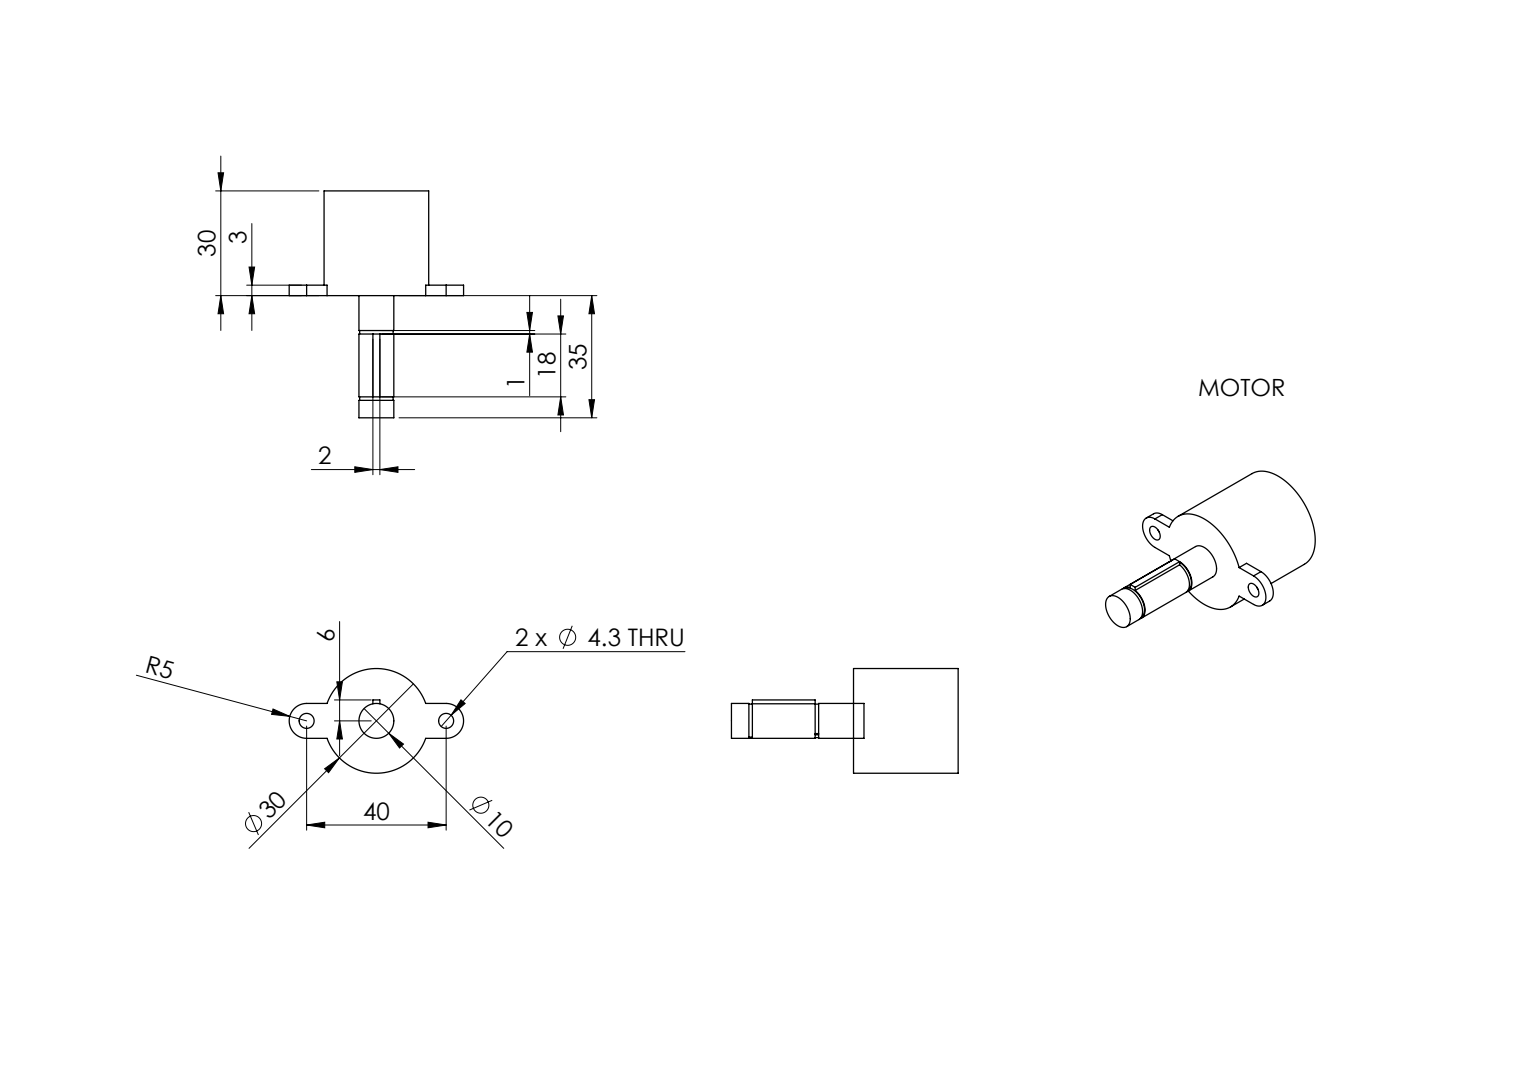
ISO-10303-21;
HEADER;
FILE_DESCRIPTION (('STEP AP214'),
    '1' );
FILE_NAME ('motor.step',
    '2026-10-31T03:44:21',
    ( '' ),
    ( '' ),
    'SwSTEP 2.0',
    'SolidWorks 2026',
    '' );
FILE_SCHEMA (( 'AUTOMOTIVE_DESIGN' ));
ENDSEC;

DATA;
#15=SURFACE_STYLE_USAGE ( .BOTH. , #11569 ) ;
#25=CARTESIAN_POINT ( 'NONE',  ( 5.000000000000003553, -20.00000000000000000, 9.999999999999998224 ) ) ;
#27=DIRECTION ( 'NONE',  ( -0.000000000000000000, -0.000000000000000000, -1.000000000000000000 ) ) ;
#44=CYLINDRICAL_SURFACE ( 'NONE', #13500, 4.799999999999999822 ) ;
#53=DIRECTION ( 'NONE',  ( -1.000000000000000000, 0.000000000000000000, 0.000000000000000000 ) ) ;
#55=CIRCLE ( 'NONE', #4760, 5.000000000000000888 ) ;
#73=CARTESIAN_POINT ( 'NONE',  ( 0.9183817310753816798, -24.91493387504114665, 15.00000000000000355 ) ) ;
#126=DIRECTION ( 'NONE',  ( -0.000000000000000000, -0.000000000000000000, -1.000000000000000000 ) ) ;
#134=ORIENTED_EDGE ( 'NONE', *, *, #5000, .T. ) ;
#135=DIRECTION ( 'NONE',  ( -9.710251638871371392E-17, -5.969973981896233748E-17, -1.000000000000000000 ) ) ;
#143=DIRECTION ( 'NONE',  ( -0.000000000000000000, -0.000000000000000000, -1.000000000000000000 ) ) ;
#149=DIRECTION ( 'NONE',  ( -0.6520673188974834833, 0.7581610723493047432, 1.805535875966851803E-17 ) ) ;
#153=VERTEX_POINT ( 'NONE', #25 ) ;
#166=CARTESIAN_POINT ( 'NONE',  ( 2.899426713160750069, -23.82535289025860337, -8.999999999999996447 ) ) ;
#171=DIRECTION ( 'NONE',  ( -0.000000000000000000, -0.000000000000000000, -1.000000000000000000 ) ) ;
#189=VERTEX_POINT ( 'NONE', #16887 ) ;
#191=ORIENTED_EDGE ( 'NONE', *, *, #16975, .F. ) ;
#195=EDGE_CURVE ( 'NONE', #14529, #9351, #3542, .T. ) ;
#218=CIRCLE ( 'NONE', #11155, 4.799999999999999822 ) ;
#226=VECTOR ( 'NONE', #4356, 1000.000000000000000 ) ;
#244=CARTESIAN_POINT ( 'NONE',  ( 22.14999999999999858, -20.00000000000000000, -20.00000000000000000 ) ) ;
#249=DIRECTION ( 'NONE',  ( -9.710251638871371392E-17, -5.969973981896233748E-17, -1.000000000000000000 ) ) ;
#257=DIRECTION ( 'NONE',  ( 0.1836763462126260738, -0.9829867750086873635, -1.521953536530129477E-22 ) ) ;
#284=ORIENTED_EDGE ( 'NONE', *, *, #7843, .F. ) ;
#301=EDGE_CURVE ( 'NONE', #4092, #18359, #6415, .T. ) ;
#302=EDGE_LOOP ( 'NONE', ( #1176, #3986, #11938, #3229 ) ) ;
#332=AXIS2_PLACEMENT_3D ( 'NONE', #14150, #12396, #6331 ) ;
#421=ORIENTED_EDGE ( 'NONE', *, *, #11100, .F. ) ;
#427=DIRECTION ( 'NONE',  ( -9.710251638871371392E-17, -5.969973981896233748E-17, -1.000000000000000000 ) ) ;
#449=CARTESIAN_POINT ( 'NONE',  ( 1.171083334267915221, -24.65495046420793201, 9.999999999999998224 ) ) ;
#461=ORIENTED_EDGE ( 'NONE', *, *, #12754, .F. ) ;
#464=VECTOR ( 'NONE', #12532, 1000.000000000000000 ) ;
#476=CARTESIAN_POINT ( 'NONE',  ( 2.449293598294706513E-15, -20.00000000000000000, -50.00000000000000000 ) ) ;
#480=CARTESIAN_POINT ( 'NONE',  ( 15.00000000000000178, -20.00000000000000000, -50.00000000000000000 ) ) ;
#484=ORIENTED_EDGE ( 'NONE', *, *, #4734, .T. ) ;
#531=CARTESIAN_POINT ( 'NONE',  ( 20.00000000000000000, -14.99999999999999289, -20.00000000000000000 ) ) ;
#541=ORIENTED_EDGE ( 'NONE', *, *, #9614, .T. ) ;
#547=AXIS2_PLACEMENT_3D ( 'NONE', #18765, #4147, #14614 ) ;
#556=ORIENTED_EDGE ( 'NONE', *, *, #7640, .F. ) ;
#557=VECTOR ( 'NONE', #8744, 1000.000000000000000 ) ;
#589=CYLINDRICAL_SURFACE ( 'NONE', #2546, 5.000000000000000888 ) ;
#603=LINE ( 'NONE', #2181, #4937 ) ;
#607=CYLINDRICAL_SURFACE ( 'NONE', #15492, 15.00000000000000000 ) ;
#614=CARTESIAN_POINT ( 'NONE',  ( 2.449293598294706513E-15, -20.00000000000000000, 15.00000000000000355 ) ) ;
#644=EDGE_CURVE ( 'NONE', #9042, #12835, #16688, .T. ) ;
#649=CIRCLE ( 'NONE', #7227, 5.000000000000007994 ) ;
#658=ADVANCED_FACE ( 'NONE', ( #13962 ), #8085, .T. ) ;
#664=CARTESIAN_POINT ( 'NONE',  ( 1.267864665261691752E-11, -20.00000000000000000, 9.999999999999998224 ) ) ;
#704=CIRCLE ( 'NONE', #1338, 5.000000000000000888 ) ;
#726=ORIENTED_EDGE ( 'NONE', *, *, #14827, .T. ) ;
#733=CARTESIAN_POINT ( 'NONE',  ( 2.899426713160750069, -23.82535289025860337, -8.999999999999996447 ) ) ;
#741=DIRECTION ( 'NONE',  ( 0.000000000000000000, 1.000000000000000000, 0.000000000000000000 ) ) ;
#781=ORIENTED_EDGE ( 'NONE', *, *, #10591, .F. ) ;
#787=EDGE_CURVE ( 'NONE', #6069, #5525, #6343, .T. ) ;
#805=LINE ( 'NONE', #17384, #2831 ) ;
#809=DIRECTION ( 'NONE',  ( 0.000000000000000000, 0.000000000000000000, -1.000000000000000000 ) ) ;
#839=DIRECTION ( 'NONE',  ( 0.000000000000000000, -0.000000000000000000, 1.000000000000000000 ) ) ;
#879=EDGE_LOOP ( 'NONE', ( #461, #556, #5752, #5214, #13460, #2512, #1411, #3266, #13006, #1930, #16328, #7538, #4298, #13725, #7198, #16875, #3831, #8695, #14190, #13668 ) ) ;
#883=EDGE_CURVE ( 'NONE', #9304, #15612, #704, .T. ) ;
#905=ADVANCED_FACE ( 'NONE', ( #9056 ), #10327, .F. ) ;
#909=AXIS2_PLACEMENT_3D ( 'NONE', #9474, #8004, #12326 ) ;
#926=VECTOR ( 'NONE', #18447, 1000.000000000000000 ) ;
#932=ORIENTED_EDGE ( 'NONE', *, *, #15552, .T. ) ;
#948=EDGE_LOOP ( 'NONE', ( #5660, #14767, #16075, #4087 ) ) ;
#953=EDGE_CURVE ( 'NONE', #5878, #5734, #2284, .T. ) ;
#967=DIRECTION ( 'NONE',  ( 9.858538378746663627E-23, -5.031452844637890958E-23, 1.000000000000000000 ) ) ;
#999=CARTESIAN_POINT ( 'NONE',  ( -4.999999999999998224, -20.00000000000000000, 15.00000000000000355 ) ) ;
#1006=ADVANCED_FACE ( 'NONE', ( #11896, #16716 ), #7399, .T. ) ;
#1036=ORIENTED_EDGE ( 'NONE', *, *, #11412, .T. ) ;
#1043=DIRECTION ( 'NONE',  ( 0.000000000000000000, 0.000000000000000000, -1.000000000000000000 ) ) ;
#1044=DIRECTION ( 'NONE',  ( -0.9697813467099857254, -0.2439756946365076173, 1.379242460255691792E-22 ) ) ;
#1056=VERTEX_POINT ( 'NONE', #15617 ) ;
#1065=EDGE_CURVE ( 'NONE', #10087, #17459, #7878, .T. ) ;
#1073=DIRECTION ( 'NONE',  ( 9.858538378746663627E-23, -5.031452844637890958E-23, 1.000000000000000000 ) ) ;
#1080=VERTEX_POINT ( 'NONE', #8056 ) ;
#1094=CARTESIAN_POINT ( 'NONE',  ( 5.000000000000003553, -20.00000000000000000, 9.000000000000000000 ) ) ;
#1096=VERTEX_POINT ( 'NONE', #9722 ) ;
#1107=CARTESIAN_POINT ( 'NONE',  ( -3.734041964264191549, -23.01611183630746638, -8.999999999999996447 ) ) ;
#1109=DIRECTION ( 'NONE',  ( 1.000000000000000000, 0.000000000000000000, 0.000000000000000000 ) ) ;
#1111=LINE ( 'NONE', #17781, #4763 ) ;
#1120=CARTESIAN_POINT ( 'NONE',  ( 2.449293598294706513E-15, -20.00000000000000000, -20.00000000000000000 ) ) ;
#1130=EDGE_CURVE ( 'NONE', #18302, #12106, #15719, .T. ) ;
#1132=DIRECTION ( 'NONE',  ( 0.000000000000000000, 0.000000000000000000, 1.000000000000000000 ) ) ;
#1152=ORIENTED_EDGE ( 'NONE', *, *, #9150, .T. ) ;
#1155=DIRECTION ( 'NONE',  ( -9.858538378746663627E-23, 5.031452844637890958E-23, -1.000000000000000000 ) ) ;
#1168=CARTESIAN_POINT ( 'NONE',  ( 1.267864665261691752E-11, -20.00000000000000000, 9.999999999999998224 ) ) ;
#1176=ORIENTED_EDGE ( 'NONE', *, *, #18527, .T. ) ;
#1179=EDGE_CURVE ( 'NONE', #8779, #4092, #13851, .T. ) ;
#1194=VECTOR ( 'NONE', #12290, 1000.000000000000000 ) ;
#1238=CIRCLE ( 'NONE', #3129, 5.000000000000000888 ) ;
#1241=ORIENTED_EDGE ( 'NONE', *, *, #11894, .T. ) ;
#1262=EDGE_CURVE ( 'NONE', #6920, #5143, #18873, .T. ) ;
#1296=( NAMED_UNIT ( * ) SI_UNIT ( $, .STERADIAN. ) SOLID_ANGLE_UNIT ( ) );
#1299=CARTESIAN_POINT ( 'NONE',  ( -20.00000000000000000, -19.99999999999999289, -20.00000000000000000 ) ) ;
#1301=DIRECTION ( 'NONE',  ( -0.9768494444668812671, -0.2139279384389642935, 0.000000000000000000 ) ) ;
#1321=VERTEX_POINT ( 'NONE', #1107 ) ;
#1338=AXIS2_PLACEMENT_3D ( 'NONE', #16043, #1132, #2717 ) ;
#1340=CARTESIAN_POINT ( 'NONE',  ( 2.449293598294706513E-15, -20.00000000000000000, 9.000000000000000000 ) ) ;
#1346=ORIENTED_EDGE ( 'NONE', *, *, #10591, .T. ) ;
#1361=ORIENTED_EDGE ( 'NONE', *, *, #9544, .T. ) ;
#1376=AXIS2_PLACEMENT_3D ( 'NONE', #10644, #15161, #18227 ) ;
#1386=( NAMED_UNIT ( * ) PLANE_ANGLE_UNIT ( ) SI_UNIT ( $, .RADIAN. ) );
#1411=ORIENTED_EDGE ( 'NONE', *, *, #17612, .T. ) ;
#1431=CARTESIAN_POINT ( 'NONE',  ( 1.219878473194463187, -24.84890673354692936, 9.000000000000000000 ) ) ;
#1433=VERTEX_POINT ( 'NONE', #19268 ) ;
#1440=CARTESIAN_POINT ( 'NONE',  ( 3.734041964264196434, -16.98388816369253362, -8.999999999999996447 ) ) ;
#1449=VECTOR ( 'NONE', #9677, 1000.000000000000000 ) ;
#1464=VERTEX_POINT ( 'NONE', #4636 ) ;
#1465=CIRCLE ( 'NONE', #3966, 5.000000000000000888 ) ;
#1515=LINE ( 'NONE', #10515, #14294 ) ;
#1537=DIRECTION ( 'NONE',  ( -9.710251638871371392E-17, -5.969973981896233748E-17, -1.000000000000000000 ) ) ;
#1540=EDGE_LOOP ( 'NONE', ( #1152, #15028, #8656, #5746 ) ) ;
#1552=AXIS2_PLACEMENT_3D ( 'NONE', #12885, #14449, #2511 ) ;
#1564=DIRECTION ( 'NONE',  ( -1.000000000000000000, 0.000000000000000000, 0.000000000000000000 ) ) ;
#1583=CIRCLE ( 'NONE', #332, 2.149999999999999023 ) ;
#1589=ORIENTED_EDGE ( 'NONE', *, *, #12157, .F. ) ;
#1620=EDGE_CURVE ( 'NONE', #6069, #8597, #7945, .T. ) ;
#1639=ORIENTED_EDGE ( 'NONE', *, *, #8427, .F. ) ;
#1640=EDGE_CURVE ( 'NONE', #7188, #13385, #11165, .T. ) ;
#1649=VERTEX_POINT ( 'NONE', #1788 ) ;
#1658=AXIS2_PLACEMENT_3D ( 'NONE', #6218, #16429, #16626 ) ;
#1684=ORIENTED_EDGE ( 'NONE', *, *, #3634, .F. ) ;
#1726=DIRECTION ( 'NONE',  ( -0.000000000000000000, -0.000000000000000000, -1.000000000000000000 ) ) ;
#1729=AXIS2_PLACEMENT_3D ( 'NONE', #5086, #9578, #3243 ) ;
#1788=CARTESIAN_POINT ( 'NONE',  ( -4.999999999999998224, -20.00000000000000000, -8.999999999999998224 ) ) ;
#1801=CIRCLE ( 'NONE', #19045, 15.00000000000000000 ) ;
#1822=LINE ( 'NONE', #7693, #18162 ) ;
#1874=AXIS2_PLACEMENT_3D ( 'NONE', #13952, #15437, #13862 ) ;
#1885=AXIS2_PLACEMENT_3D ( 'NONE', #2595, #11864, #19063 ) ;
#1898=CARTESIAN_POINT ( 'NONE',  ( -4.999999999999998224, -20.00000000000000000, 9.000000000000000000 ) ) ;
#1908=EDGE_CURVE ( 'NONE', #2621, #7384, #4316, .T. ) ;
#1925=CARTESIAN_POINT ( 'NONE',  ( -4.999999999999998224, -20.00000000000000000, 15.00000000000000355 ) ) ;
#1930=ORIENTED_EDGE ( 'NONE', *, *, #7858, .T. ) ;
#1983=CYLINDRICAL_SURFACE ( 'NONE', #3497, 5.000000000000000888 ) ;
#1994=DIRECTION ( 'NONE',  ( -1.000000000000000000, 0.000000000000000000, 0.000000000000000000 ) ) ;
#2014=ORIENTED_EDGE ( 'NONE', *, *, #18527, .F. ) ;
#2023=LINE ( 'NONE', #449, #17601 ) ;
#2049=EDGE_LOOP ( 'NONE', ( #1684, #9569, #5626, #12124, #5368, #18796, #18625, #17262 ) ) ;
#2056=CIRCLE ( 'NONE', #18350, 4.799999999999999822 ) ;
#2059=ORIENTED_EDGE ( 'NONE', *, *, #953, .F. ) ;
#2075=CARTESIAN_POINT ( 'NONE',  ( 2.449293598294706513E-15, -20.00000000000000000, 15.00000000000000355 ) ) ;
#2095=EDGE_CURVE ( 'NONE', #2791, #16221, #9204, .T. ) ;
#2097=CARTESIAN_POINT ( 'NONE',  ( -0.9999999999999976685, -20.00000000000000000, 8.999999999999998224 ) ) ;
#2114=DIRECTION ( 'NONE',  ( -9.710251638871371392E-17, -5.969973981896233748E-17, -1.000000000000000000 ) ) ;
#2117=CYLINDRICAL_SURFACE ( 'NONE', #15082, 2.149999999999999023 ) ;
#2131=ADVANCED_FACE ( 'NONE', ( #3523 ), #16968, .F. ) ;
#2139=( NAMED_UNIT ( * ) PLANE_ANGLE_UNIT ( ) SI_UNIT ( $, .RADIAN. ) );
#2141=ORIENTED_EDGE ( 'NONE', *, *, #15552, .F. ) ;
#2167=ORIENTED_EDGE ( 'NONE', *, *, #12021, .F. ) ;
#2170=CARTESIAN_POINT ( 'NONE',  ( 15.00000000000000178, -20.00000000000000000, -50.00000000000000000 ) ) ;
#2172=DIRECTION ( 'NONE',  ( 1.000000000000000000, 0.000000000000000000, 0.000000000000000000 ) ) ;
#2178=CIRCLE ( 'NONE', #2497, 4.800000000000000711 ) ;
#2181=CARTESIAN_POINT ( 'NONE',  ( 5.000000000000003553, -20.00000000000000000, 15.00000000000000355 ) ) ;
#2189=AXIS2_PLACEMENT_3D ( 'NONE', #14814, #14713, #1301 ) ;
#2193=DIRECTION ( 'NONE',  ( 0.000000000000000000, 0.000000000000000000, 1.000000000000000000 ) ) ;
#2208=EDGE_CURVE ( 'NONE', #17459, #7605, #2451, .T. ) ;
#2209=ORIENTED_EDGE ( 'NONE', *, *, #1620, .F. ) ;
#2246=VECTOR ( 'NONE', #6356, 1000.000000000000000 ) ;
#2254=VERTEX_POINT ( 'NONE', #5566 ) ;
#2281=DIRECTION ( 'NONE',  ( 0.000000000000000000, 0.000000000000000000, 1.000000000000000000 ) ) ;
#2284=CIRCLE ( 'NONE', #8215, 2.149999999999999023 ) ;
#2297=FACE_OUTER_BOUND ( 'NONE', #18445, .T. ) ;
#2341=EDGE_CURVE ( 'NONE', #1056, #14529, #13510, .T. ) ;
#2342=DIRECTION ( 'NONE',  ( 0.000000000000000000, 0.000000000000000000, -1.000000000000000000 ) ) ;
#2348=ORIENTED_EDGE ( 'NONE', *, *, #18323, .F. ) ;
#2355=CARTESIAN_POINT ( 'NONE',  ( 2.385244779468109755E-15, -20.00000000000000000, -9.999999999999994671 ) ) ;
#2370=AXIS2_PLACEMENT_3D ( 'NONE', #8722, #12053, #16478 ) ;
#2401=LINE ( 'NONE', #5416, #10995 ) ;
#2418=ORIENTED_EDGE ( 'NONE', *, *, #18926, .T. ) ;
#2426=PLANE ( 'NONE',  #11494 ) ;
#2431=VECTOR ( 'NONE', #5881, 1000.000000000000000 ) ;
#2451=LINE ( 'NONE', #2653, #1449 ) ;
#2453=VECTOR ( 'NONE', #15403, 999.9999999999998863 ) ;
#2497=AXIS2_PLACEMENT_3D ( 'NONE', #18498, #18305, #16731 ) ;
#2511=DIRECTION ( 'NONE',  ( 1.000000000000000000, -1.734723475976807341E-16, 0.000000000000000000 ) ) ;
#2512=ORIENTED_EDGE ( 'NONE', *, *, #12998, .T. ) ;
#2526=EDGE_CURVE ( 'NONE', #5878, #8101, #2401, .T. ) ;
#2546=AXIS2_PLACEMENT_3D ( 'NONE', #3628, #18454, #14567 ) ;
#2550=AXIS2_PLACEMENT_3D ( 'NONE', #3299, #15637, #15439 ) ;
#2553=LINE ( 'NONE', #14672, #17765 ) ;
#2556=FACE_OUTER_BOUND ( 'NONE', #16354, .T. ) ;
#2569=LINE ( 'NONE', #14496, #4883 ) ;
#2586=EDGE_CURVE ( 'NONE', #189, #17705, #1111, .T. ) ;
#2595=CARTESIAN_POINT ( 'NONE',  ( 1.267864665261691752E-11, -20.00000000000000000, 9.999999999999998224 ) ) ;
#2621=VERTEX_POINT ( 'NONE', #6983 ) ;
#2627=CARTESIAN_POINT ( 'NONE',  ( 3.129923130707922496, -23.63917314727666152, -8.999999999999996447 ) ) ;
#2650=CARTESIAN_POINT ( 'NONE',  ( 20.00000000000000000, -20.00000000000000000, -20.00000000000000000 ) ) ;
#2652=DIRECTION ( 'NONE',  ( -0.7779254092217071648, -0.6283566325640553840, 0.000000000000000000 ) ) ;
#2653=CARTESIAN_POINT ( 'NONE',  ( -1.000000000000000000, -14.00000000000000000, 8.999999999999998224 ) ) ;
#2683=VECTOR ( 'NONE', #17447, 1000.000000000000000 ) ;
#2687=CARTESIAN_POINT ( 'NONE',  ( 20.00000000000000000, -20.00000000000000000, -23.00000000000000000 ) ) ;
#2696=EDGE_CURVE ( 'NONE', #7605, #9351, #4641, .T. ) ;
#2707=DIRECTION ( 'NONE',  ( 0.000000000000000000, 0.000000000000000000, -1.000000000000000000 ) ) ;
#2712=CARTESIAN_POINT ( 'NONE',  ( -4.688877333428353111, -21.02685410450703074, 9.999999999999998224 ) ) ;
#2717=DIRECTION ( 'NONE',  ( 1.000000000000000000, 0.000000000000000000, 0.000000000000000000 ) ) ;
#2745=DIRECTION ( 'NONE',  ( -4.082155997157844188E-16, 1.000000000000000000, 0.000000000000000000 ) ) ;
#2763=EDGE_CURVE ( 'NONE', #12835, #6920, #3511, .T. ) ;
#2764=AXIS2_PLACEMENT_3D ( 'NONE', #9423, #9512, #6382 ) ;
#2771=CARTESIAN_POINT ( 'NONE',  ( 2.449293598294706513E-15, -20.00000000000000000, -23.00000000000000000 ) ) ;
#2773=VECTOR ( 'NONE', #14133, 1000.000000000000000 ) ;
#2775=LINE ( 'NONE', #17768, #7973 ) ;
#2777=CYLINDRICAL_SURFACE ( 'NONE', #1885, 4.800000000000000711 ) ;
#2791=VERTEX_POINT ( 'NONE', #2170 ) ;
#2831=VECTOR ( 'NONE', #18960, 1000.000000000000000 ) ;
#2834=FACE_OUTER_BOUND ( 'NONE', #7295, .T. ) ;
#2841=EDGE_CURVE ( 'NONE', #7251, #10053, #7325, .T. ) ;
#2856=UNCERTAINTY_MEASURE_WITH_UNIT (LENGTH_MEASURE( 1.000000000000000082E-05 ), #11966, 'distance_accuracy_value', 'NONE');
#2857=CARTESIAN_POINT ( 'NONE',  ( 4.688877333453708829, -18.97314589549297281, 9.999999999999998224 ) ) ;
#2871=CARTESIAN_POINT ( 'NONE',  ( 0.000000000000000000, 0.000000000000000000, 0.000000000000000000 ) ) ;
#2893=EDGE_LOOP ( 'NONE', ( #14519, #1241, #8781, #541, #15083, #16639, #1361, #2418, #6160, #17930, #16178, #3967 ) ) ;
#2961=EDGE_CURVE ( 'NONE', #10552, #3811, #14966, .T. ) ;
#2963=FILL_AREA_STYLE ('',( #16396 ) ) ;
#2992=DIRECTION ( 'NONE',  ( -4.082155997157844188E-16, 1.000000000000000000, 0.000000000000000000 ) ) ;
#2996=EDGE_CURVE ( 'NONE', #8876, #2621, #15399, .T. ) ;
#3026=DIRECTION ( 'NONE',  ( -1.000000000000000000, 0.000000000000000000, 0.000000000000000000 ) ) ;
#3029=ORIENTED_EDGE ( 'NONE', *, *, #7729, .T. ) ;
#3050=CLOSED_SHELL ( 'NONE', ( #11551, #12818, #12677, #16496, #16720, #7692, #5212, #9043, #16819, #4658, #7547, #13586, #5565, #10107, #11468, #16105, #7593, #15278, #14470, #2131, #1006, #14914, #5238, #17940, #13003, #905, #6926, #658, #10337, #18770, #8668, #8209, #4637, #10878, #8572, #15621, #16901, #15242, #8795, #15598 ) ) ;
#3097=AXIS2_PLACEMENT_3D ( 'NONE', #13122, #9094, #19329 ) ;
#3107=ORIENTED_EDGE ( 'NONE', *, *, #2341, .F. ) ;
#3125=LINE ( 'NONE', #15355, #8048 ) ;
#3128=AXIS2_PLACEMENT_3D ( 'NONE', #1120, #2707, #13075 ) ;
#3129=AXIS2_PLACEMENT_3D ( 'NONE', #1340, #7313, #10147 ) ;
#3134=ORIENTED_EDGE ( 'NONE', *, *, #15693, .T. ) ;
#3145=DIRECTION ( 'NONE',  ( -0.7779254092217071648, -0.6283566325640553840, 0.000000000000000000 ) ) ;
#3196=AXIS2_PLACEMENT_3D ( 'NONE', #10224, #4259, #4072 ) ;
#3200=VECTOR ( 'NONE', #2745, 1000.000000000000000 ) ;
#3204=ORIENTED_EDGE ( 'NONE', *, *, #4625, .F. ) ;
#3208=EDGE_LOOP ( 'NONE', ( #4399, #3539, #9450, #15588 ) ) ;
#3212=PLANE ( 'NONE',  #13485 ) ;
#3229=ORIENTED_EDGE ( 'NONE', *, *, #17743, .F. ) ;
#3240=LINE ( 'NONE', #12050, #13687 ) ;
#3243=DIRECTION ( 'NONE',  ( -0.7779254092217071648, -0.6283566325640553840, 1.130512422757410748E-16 ) ) ;
#3266=ORIENTED_EDGE ( 'NONE', *, *, #10585, .F. ) ;
#3278=CARTESIAN_POINT ( 'NONE',  ( 17.85000000000000142, -20.00000000000000000, -20.00000000000000000 ) ) ;
#3285=DIRECTION ( 'NONE',  ( -1.000000000000000000, 0.000000000000000000, -0.000000000000000000 ) ) ;
#3299=CARTESIAN_POINT ( 'NONE',  ( 2.449293598294706513E-15, -20.00000000000000000, -23.00000000000000000 ) ) ;
#3302=PLANE ( 'NONE',  #15384 ) ;
#3326=VERTEX_POINT ( 'NONE', #11798 ) ;
#3346=AXIS2_PLACEMENT_3D ( 'NONE', #614, #7962, #15717 ) ;
#3360=FACE_OUTER_BOUND ( 'NONE', #8105, .T. ) ;
#3369=ORIENTED_EDGE ( 'NONE', *, *, #14240, .T. ) ;
#3417=ORIENTED_EDGE ( 'NONE', *, *, #11894, .F. ) ;
#3422=AXIS2_PLACEMENT_3D ( 'NONE', #664, #16952, #15176 ) ;
#3447=VECTOR ( 'NONE', #15223, 1000.000000000000000 ) ;
#3475=DIRECTION ( 'NONE',  ( -0.000000000000000000, -0.000000000000000000, 1.000000000000000000 ) ) ;
#3494=VECTOR ( 'NONE', #257, 999.9999999999998863 ) ;
#3497=AXIS2_PLACEMENT_3D ( 'NONE', #2075, #14115, #9598 ) ;
#3511=CIRCLE ( 'NONE', #13533, 5.000000000000000888 ) ;
#3515=ORIENTED_EDGE ( 'NONE', *, *, #14193, .F. ) ;
#3523=FACE_OUTER_BOUND ( 'NONE', #11989, .T. ) ;
#3528=ORIENTED_EDGE ( 'NONE', *, *, #7944, .F. ) ;
#3539=ORIENTED_EDGE ( 'NONE', *, *, #10524, .F. ) ;
#3542=LINE ( 'NONE', #9314, #9848 ) ;
#3579=ORIENTED_EDGE ( 'NONE', *, *, #883, .T. ) ;
#3607=ORIENTED_EDGE ( 'NONE', *, *, #10362, .F. ) ;
#3628=CARTESIAN_POINT ( 'NONE',  ( 2.449293598294706513E-15, -20.00000000000000000, 15.00000000000000355 ) ) ;
#3634=EDGE_CURVE ( 'NONE', #1433, #2791, #19259, .T. ) ;
#3645=CARTESIAN_POINT ( 'NONE',  ( 1.000000000000000000, -14.00000000000000000, 8.999999999999998224 ) ) ;
#3647=CARTESIAN_POINT ( 'NONE',  ( 2.449293598294706513E-15, -20.00000000000000000, -50.00000000000000000 ) ) ;
#3656=FACE_OUTER_BOUND ( 'NONE', #1540, .T. ) ;
#3712=CARTESIAN_POINT ( 'NONE',  ( 2.449293598294706513E-15, -20.00000000000000000, 15.00000000000000355 ) ) ;
#3737=VECTOR ( 'NONE', #14659, 1000.000000000000000 ) ;
#3797=CARTESIAN_POINT ( 'NONE',  ( 2.482347295856823136E-15, -20.00000000000000000, -8.999999999999996447 ) ) ;
#3811=VERTEX_POINT ( 'NONE', #11480 ) ;
#3820=EDGE_CURVE ( 'NONE', #1464, #8101, #12968, .T. ) ;
#3829=CARTESIAN_POINT ( 'NONE',  ( 2.482347295856823136E-15, -20.00000000000000000, -8.999999999999996447 ) ) ;
#3831=ORIENTED_EDGE ( 'NONE', *, *, #9143, .F. ) ;
#3864=EDGE_LOOP ( 'NONE', ( #6325, #14684, #12211, #4511 ) ) ;
#3870=ORIENTED_EDGE ( 'NONE', *, *, #1130, .T. ) ;
#3891=EDGE_LOOP ( 'NONE', ( #12395, #17263 ) ) ;
#3911=CARTESIAN_POINT ( 'NONE',  ( 3.020236159542450949, -23.98474259401938014, 15.00000000000000355 ) ) ;
#3943=DIRECTION ( 'NONE',  ( -1.000000000000000000, 0.000000000000000000, 0.000000000000000000 ) ) ;
#3963=CARTESIAN_POINT ( 'NONE',  ( -1.000000000000000000, -14.00000000000000000, -9.000000000000001776 ) ) ;
#3966=AXIS2_PLACEMENT_3D ( 'NONE', #14131, #2193, #6784 ) ;
#3967=ORIENTED_EDGE ( 'NONE', *, *, #195, .T. ) ;
#3986=ORIENTED_EDGE ( 'NONE', *, *, #14771, .F. ) ;
#3991=FACE_OUTER_BOUND ( 'NONE', #16059, .T. ) ;
#4040=ORIENTED_EDGE ( 'NONE', *, *, #15055, .F. ) ;
#4050=EDGE_CURVE ( 'NONE', #1649, #1056, #16119, .T. ) ;
#4063=EDGE_LOOP ( 'NONE', ( #8392, #17053 ) ) ;
#4072=DIRECTION ( 'NONE',  ( -1.000000000000000000, 0.000000000000000000, 0.000000000000000000 ) ) ;
#4087=ORIENTED_EDGE ( 'NONE', *, *, #4050, .F. ) ;
#4092=VERTEX_POINT ( 'NONE', #18267 ) ;
#4147=DIRECTION ( 'NONE',  ( 0.000000000000000000, 0.000000000000000000, -1.000000000000000000 ) ) ;
#4212=CARTESIAN_POINT ( 'NONE',  ( 4.688877333453707941, -18.97314589549297281, 9.999999999999998224 ) ) ;
#4215=CARTESIAN_POINT ( 'NONE',  ( 0.9183817310753817909, -24.91493387504115020, 9.000000000000000000 ) ) ;
#4259=DIRECTION ( 'NONE',  ( -9.710251638871371392E-17, -5.969973981896233748E-17, -1.000000000000000000 ) ) ;
#4298=ORIENTED_EDGE ( 'NONE', *, *, #1908, .F. ) ;
#4316=LINE ( 'NONE', #10285, #11766 ) ;
#4325=( LENGTH_UNIT ( ) NAMED_UNIT ( * ) SI_UNIT ( .MILLI., .METRE. ) );
#4331=DIRECTION ( 'NONE',  ( -0.000000000000000000, -0.000000000000000000, 1.000000000000000000 ) ) ;
#4356=DIRECTION ( 'NONE',  ( -0.000000000000000000, -0.000000000000000000, 1.000000000000000000 ) ) ;
#4360=EDGE_CURVE ( 'NONE', #1080, #13316, #7668, .T. ) ;
#4364=FACE_OUTER_BOUND ( 'NONE', #302, .T. ) ;
#4382=EDGE_LOOP ( 'NONE', ( #17344, #13774 ) ) ;
#4387=VERTEX_POINT ( 'NONE', #4215 ) ;
#4399=ORIENTED_EDGE ( 'NONE', *, *, #2526, .F. ) ;
#4455=ORIENTED_EDGE ( 'NONE', *, *, #14348, .F. ) ;
#4457=DIRECTION ( 'NONE',  ( 0.000000000000000000, 0.000000000000000000, -1.000000000000000000 ) ) ;
#4508=DIRECTION ( 'NONE',  ( -0.000000000000000000, -0.000000000000000000, 1.000000000000000000 ) ) ;
#4511=ORIENTED_EDGE ( 'NONE', *, *, #2696, .T. ) ;
#4550=AXIS2_PLACEMENT_3D ( 'NONE', #18472, #249, #12663 ) ;
#4559=CARTESIAN_POINT ( 'NONE',  ( 5.000000000000003553, -20.00000000000000000, -20.00000000000000000 ) ) ;
#4589=CARTESIAN_POINT ( 'NONE',  ( -20.00000000000000000, -25.00000000000000000, -20.00000000000000000 ) ) ;
#4625=EDGE_CURVE ( 'NONE', #15442, #4903, #13987, .T. ) ;
#4636=CARTESIAN_POINT ( 'NONE',  ( -22.14999999999999858, -19.99999999999999289, -23.00000000000000000 ) ) ;
#4637=ADVANCED_FACE ( 'NONE', ( #4711 ), #18543, .F. ) ;
#4641=LINE ( 'NONE', #11876, #15387 ) ;
#4656=VECTOR ( 'NONE', #4508, 1000.000000000000000 ) ;
#4658=ADVANCED_FACE ( 'NONE', ( #2556 ), #11537, .T. ) ;
#4672=MECHANICAL_DESIGN_GEOMETRIC_PRESENTATION_REPRESENTATION('',(#4964),#8404);
#4711=FACE_OUTER_BOUND ( 'NONE', #9286, .T. ) ;
#4717=VECTOR ( 'NONE', #1537, 1000.000000000000000 ) ;
#4734=EDGE_CURVE ( 'NONE', #6996, #18140, #12051, .T. ) ;
#4749=EDGE_CURVE ( 'NONE', #18696, #18359, #18831, .T. ) ;
#4760=AXIS2_PLACEMENT_3D ( 'NONE', #11167, #2281, #16993 ) ;
#4763=VECTOR ( 'NONE', #17399, 1000.000000000000000 ) ;
#4765=CARTESIAN_POINT ( 'NONE',  ( 0.000000000000000000, 0.000000000000000000, -9.000000000000001776 ) ) ;
#4775=CARTESIAN_POINT ( 'NONE',  ( 0.8816464618332836567, -24.71833652004169934, 9.000000000000000000 ) ) ;
#4787=EDGE_LOOP ( 'NONE', ( #8005, #10366, #16026, #5421 ) ) ;
#4834=CARTESIAN_POINT ( 'NONE',  ( 15.00000000000000178, -20.00000000000000000, -23.00000000000000000 ) ) ;
#4836=EDGE_CURVE ( 'NONE', #12060, #13420, #17254, .T. ) ;
#4841=FACE_OUTER_BOUND ( 'NONE', #11042, .T. ) ;
#4863=CARTESIAN_POINT ( 'NONE',  ( 2.449293598294706513E-15, -20.00000000000000000, -8.999999999999998224 ) ) ;
#4883=VECTOR ( 'NONE', #14788, 999.9999999999998863 ) ;
#4885=( NAMED_UNIT ( * ) SI_UNIT ( $, .STERADIAN. ) SOLID_ANGLE_UNIT ( ) );
#4903=VERTEX_POINT ( 'NONE', #4589 ) ;
#4904=LINE ( 'NONE', #10871, #13097 ) ;
#4928=VERTEX_POINT ( 'NONE', #11638 ) ;
#4933=CARTESIAN_POINT ( 'NONE',  ( -4.999999999999998224, -20.00000000000000000, -9.999999999999994671 ) ) ;
#4937=VECTOR ( 'NONE', #10888, 1000.000000000000000 ) ;
#4944=DIRECTION ( 'NONE',  ( -1.000000000000000000, 0.000000000000000000, 0.000000000000000000 ) ) ;
#4964=STYLED_ITEM('',(#19482),#15206);
#4986=DIRECTION ( 'NONE',  ( -1.000000000000000000, 1.734723475976806848E-16, 0.000000000000000000 ) ) ;
#4992=AXIS2_PLACEMENT_3D ( 'NONE', #12281, #18281, #1994 ) ;
#5000=EDGE_CURVE ( 'NONE', #15442, #189, #17049, .T. ) ;
#5029=CARTESIAN_POINT ( 'NONE',  ( 2.482347295856823136E-15, -20.00000000000000000, -8.999999999999996447 ) ) ;
#5050=ORIENTED_EDGE ( 'NONE', *, *, #11929, .F. ) ;
#5073=VERTEX_POINT ( 'NONE', #15721 ) ;
#5086=CARTESIAN_POINT ( 'NONE',  ( 2.385244779468109755E-15, -20.00000000000000000, -9.999999999999994671 ) ) ;
#5088=CARTESIAN_POINT ( 'NONE',  ( -14.14213562373094568, -14.99999999999998757, -20.00000000000000000 ) ) ;
#5094=DIRECTION ( 'NONE',  ( -1.000000000000000000, 0.000000000000000000, 0.000000000000000000 ) ) ;
#5118=LINE ( 'NONE', #17097, #17763 ) ;
#5120=LINE ( 'NONE', #9434, #10842 ) ;
#5143=VERTEX_POINT ( 'NONE', #5220 ) ;
#5145=AXIS2_PLACEMENT_3D ( 'NONE', #17979, #27, #8742 ) ;
#5156=AXIS2_PLACEMENT_3D ( 'NONE', #10694, #12353, #11071 ) ;
#5166=CARTESIAN_POINT ( 'NONE',  ( 20.00000000000000000, -25.00000000000000711, -23.00000000000000000 ) ) ;
#5170=LINE ( 'NONE', #11142, #10219 ) ;
#5212=ADVANCED_FACE ( 'NONE', ( #17396 ), #17598, .T. ) ;
#5214=ORIENTED_EDGE ( 'NONE', *, *, #13247, .F. ) ;
#5220=CARTESIAN_POINT ( 'NONE',  ( 1.171083334267915221, -24.65495046420793201, 9.000000000000000000 ) ) ;
#5226=CIRCLE ( 'NONE', #547, 2.149999999999999023 ) ;
#5238=ADVANCED_FACE ( 'NONE', ( #14523 ), #15915, .F. ) ;
#5240=ORIENTED_EDGE ( 'NONE', *, *, #15055, .T. ) ;
#5275=AXIS2_PLACEMENT_3D ( 'NONE', #1168, #1073, #7042 ) ;
#5299=LINE ( 'NONE', #999, #11197 ) ;
#5307=CARTESIAN_POINT ( 'NONE',  ( 2.449293598294706513E-15, -20.00000000000000000, -20.00000000000000000 ) ) ;
#5324=DIRECTION ( 'NONE',  ( 0.000000000000000000, 0.000000000000000000, 1.000000000000000000 ) ) ;
#5339=ORIENTED_EDGE ( 'NONE', *, *, #2841, .F. ) ;
#5349=DIRECTION ( 'NONE',  ( -1.000000000000000000, 0.000000000000000000, 0.000000000000000000 ) ) ;
#5368=ORIENTED_EDGE ( 'NONE', *, *, #16233, .T. ) ;
#5390=CARTESIAN_POINT ( 'NONE',  ( 14.14213562373095101, -25.00000000000000711, -20.00000000000000000 ) ) ;
#5404=CARTESIAN_POINT ( 'NONE',  ( 2.449293598294706513E-15, -20.00000000000000000, 9.999999999999998224 ) ) ;
#5407=CARTESIAN_POINT ( 'NONE',  ( 2.449293598294706513E-15, -20.00000000000000000, -20.00000000000000000 ) ) ;
#5408=ORIENTED_EDGE ( 'NONE', *, *, #15044, .T. ) ;
#5416=CARTESIAN_POINT ( 'NONE',  ( -17.85000000000000142, -19.99999999999999289, -23.00000000000000000 ) ) ;
#5421=ORIENTED_EDGE ( 'NONE', *, *, #8050, .T. ) ;
#5443=LINE ( 'NONE', #11421, #17890 ) ;
#5495=DIRECTION ( 'NONE',  ( -1.000000000000000000, 0.000000000000000000, 0.000000000000000000 ) ) ;
#5525=VERTEX_POINT ( 'NONE', #18179 ) ;
#5554=ORIENTED_EDGE ( 'NONE', *, *, #3634, .T. ) ;
#5565=ADVANCED_FACE ( 'NONE', ( #12453 ), #1983, .T. ) ;
#5566=CARTESIAN_POINT ( 'NONE',  ( 14.14213562373095101, -25.00000000000000711, -23.00000000000000000 ) ) ;
#5577=PLANE ( 'NONE',  #10588 ) ;
#5599=EDGE_CURVE ( 'NONE', #7384, #9761, #55, .T. ) ;
#5624=AXIS2_PLACEMENT_3D ( 'NONE', #5404, #15905, #10996 ) ;
#5626=ORIENTED_EDGE ( 'NONE', *, *, #4360, .T. ) ;
#5650=CARTESIAN_POINT ( 'NONE',  ( 0.8816464618332836567, -24.71833652004169934, 9.999999999999998224 ) ) ;
#5660=ORIENTED_EDGE ( 'NONE', *, *, #17612, .F. ) ;
#5724=ORIENTED_EDGE ( 'NONE', *, *, #644, .T. ) ;
#5734=VERTEX_POINT ( 'NONE', #16185 ) ;
#5746=ORIENTED_EDGE ( 'NONE', *, *, #4625, .T. ) ;
#5750=DIRECTION ( 'NONE',  ( -9.858538378746663627E-23, 5.031452844637890958E-23, -1.000000000000000000 ) ) ;
#5752=ORIENTED_EDGE ( 'NONE', *, *, #8061, .T. ) ;
#5759=AXIS2_PLACEMENT_3D ( 'NONE', #8457, #11684, #7279 ) ;
#5760=DIRECTION ( 'NONE',  ( -0.000000000000000000, -0.000000000000000000, 1.000000000000000000 ) ) ;
#5798=DIRECTION ( 'NONE',  ( -0.000000000000000000, -0.000000000000000000, -1.000000000000000000 ) ) ;
#5841=ORIENTED_EDGE ( 'NONE', *, *, #15145, .F. ) ;
#5850=LINE ( 'NONE', #1440, #4717 ) ;
#5854=CARTESIAN_POINT ( 'NONE',  ( 2.449293598294706513E-15, -20.00000000000000000, -50.00000000000000000 ) ) ;
#5878=VERTEX_POINT ( 'NONE', #6085 ) ;
#5881=DIRECTION ( 'NONE',  ( -9.858538378746663627E-23, 5.031452844637890958E-23, -1.000000000000000000 ) ) ;
#5921=FACE_OUTER_BOUND ( 'NONE', #11880, .T. ) ;
#5922=ADVANCED_BREP_SHAPE_REPRESENTATION ( '', ( #15206, #10359 ), #13801 ) ;
#5935=DIRECTION ( 'NONE',  ( 0.000000000000000000, 0.000000000000000000, -1.000000000000000000 ) ) ;
#5962=DIRECTION ( 'NONE',  ( 0.000000000000000000, 0.000000000000000000, 1.000000000000000000 ) ) ;
#5975=CARTESIAN_POINT ( 'NONE',  ( 14.14213562373094923, -14.99999999999999112, -50.00000000000000000 ) ) ;
#5981=ORIENTED_EDGE ( 'NONE', *, *, #1262, .F. ) ;
#5983=ORIENTED_EDGE ( 'NONE', *, *, #11667, .F. ) ;
#6004=PRESENTATION_STYLE_ASSIGNMENT (( #15 ) ) ;
#6069=VERTEX_POINT ( 'NONE', #12534 ) ;
#6085=CARTESIAN_POINT ( 'NONE',  ( -17.85000000000000142, -19.99999999999999289, -20.00000000000000000 ) ) ;
#6154=VERTEX_POINT ( 'NONE', #5088 ) ;
#6160=ORIENTED_EDGE ( 'NONE', *, *, #10585, .T. ) ;
#6186=DIRECTION ( 'NONE',  ( -1.000000000000000000, 0.000000000000000000, 0.000000000000000000 ) ) ;
#6194=CIRCLE ( 'NONE', #9303, 2.149999999999999023 ) ;
#6210=DIRECTION ( 'NONE',  ( -9.710251638871371392E-17, -5.969973981896233748E-17, -1.000000000000000000 ) ) ;
#6218=CARTESIAN_POINT ( 'NONE',  ( 1.000000000000002442, -20.00000000000000000, 8.999999999999998224 ) ) ;
#6231=FACE_OUTER_BOUND ( 'NONE', #2049, .T. ) ;
#6237=LINE ( 'NONE', #4775, #3494 ) ;
#6255=ORIENTED_EDGE ( 'NONE', *, *, #2996, .T. ) ;
#6312=CARTESIAN_POINT ( 'NONE',  ( 20.00000000000000000, -14.99999999999999289, -23.00000000000000000 ) ) ;
#6325=ORIENTED_EDGE ( 'NONE', *, *, #195, .F. ) ;
#6331=DIRECTION ( 'NONE',  ( -1.000000000000000000, 0.000000000000000000, 0.000000000000000000 ) ) ;
#6343=CIRCLE ( 'NONE', #12284, 5.000000000000007994 ) ;
#6356=DIRECTION ( 'NONE',  ( -0.000000000000000000, -0.000000000000000000, -1.000000000000000000 ) ) ;
#6365=ORIENTED_EDGE ( 'NONE', *, *, #1262, .T. ) ;
#6382=DIRECTION ( 'NONE',  ( -0.9768494444668812671, -0.2139279384389642935, 0.000000000000000000 ) ) ;
#6400=CARTESIAN_POINT ( 'NONE',  ( -14.14213562373094746, -25.00000000000000000, -50.00000000000000000 ) ) ;
#6409=EDGE_LOOP ( 'NONE', ( #7699, #3579 ) ) ;
#6411=VERTEX_POINT ( 'NONE', #17738 ) ;
#6415=CIRCLE ( 'NONE', #5156, 2.149999999999999023 ) ;
#6470=AXIS2_PLACEMENT_3D ( 'NONE', #10421, #6210, #8953 ) ;
#6474=CIRCLE ( 'NONE', #16202, 4.799999999999999822 ) ;
#6487=CYLINDRICAL_SURFACE ( 'NONE', #3346, 5.000000000000000888 ) ;
#6514=DIRECTION ( 'NONE',  ( -0.2439756946365075896, 0.9697813467099857254, 1.610118993450814692E-22 ) ) ;
#6529=ORIENTED_EDGE ( 'NONE', *, *, #2526, .T. ) ;
#6533=CYLINDRICAL_SURFACE ( 'NONE', #3422, 4.800000000000000711 ) ;
#6548=CARTESIAN_POINT ( 'NONE',  ( -20.00000000000000000, -25.00000000000000000, -23.00000000000000000 ) ) ;
#6552=ORIENTED_EDGE ( 'NONE', *, *, #8309, .F. ) ;
#6553=VERTEX_POINT ( 'NONE', #10652 ) ;
#6562=FACE_OUTER_BOUND ( 'NONE', #11946, .T. ) ;
#6605=ORIENTED_EDGE ( 'NONE', *, *, #2208, .F. ) ;
#6616=CIRCLE ( 'NONE', #3196, 5.000000000000000888 ) ;
#6631=ORIENTED_EDGE ( 'NONE', *, *, #12754, .T. ) ;
#6635=VECTOR ( 'NONE', #12020, 1000.000000000000000 ) ;
#6639=ORIENTED_EDGE ( 'NONE', *, *, #787, .F. ) ;
#6709=CARTESIAN_POINT ( 'NONE',  ( -20.00000000000000000, -19.99999999999999289, -23.00000000000000000 ) ) ;
#6721=DIRECTION ( 'NONE',  ( -0.7779254092217071648, -0.6283566325640553840, 0.000000000000000000 ) ) ;
#6726=AXIS2_PLACEMENT_3D ( 'NONE', #2355, #9872, #2652 ) ;
#6728=DIRECTION ( 'NONE',  ( -0.7779254092217071648, -0.6283566325640553840, 0.000000000000000000 ) ) ;
#6738=DIRECTION ( 'NONE',  ( -0.000000000000000000, -0.000000000000000000, -1.000000000000000000 ) ) ;
#6754=EDGE_CURVE ( 'NONE', #12106, #4903, #5443, .T. ) ;
#6775=ORIENTED_EDGE ( 'NONE', *, *, #2841, .T. ) ;
#6784=DIRECTION ( 'NONE',  ( 1.000000000000000000, 0.000000000000000000, 0.000000000000000000 ) ) ;
#6798=AXIS2_PLACEMENT_3D ( 'NONE', #2627, #7305, #14746 ) ;
#6812=AXIS2_PLACEMENT_3D ( 'NONE', #15705, #10101, #5495 ) ;
#6821=ORIENTED_EDGE ( 'NONE', *, *, #2586, .T. ) ;
#6838=DIRECTION ( 'NONE',  ( -1.000000000000000000, 0.000000000000000000, 0.000000000000000000 ) ) ;
#6860=AXIS2_PLACEMENT_3D ( 'NONE', #14836, #4457, #14735 ) ;
#6868=DIRECTION ( 'NONE',  ( 1.000000000000000000, 0.000000000000000000, 0.000000000000000000 ) ) ;
#6891=LINE ( 'NONE', #12879, #18829 ) ;
#6910=CARTESIAN_POINT ( 'NONE',  ( 20.00000000000000000, -20.00000000000000000, -23.00000000000000000 ) ) ;
#6920=VERTEX_POINT ( 'NONE', #1431 ) ;
#6926=ADVANCED_FACE ( 'NONE', ( #11902 ), #17912, .T. ) ;
#6951=FACE_OUTER_BOUND ( 'NONE', #14837, .T. ) ;
#6957=CARTESIAN_POINT ( 'NONE',  ( -1.000000000000000000, -14.00000000000000000, 8.999999999999998224 ) ) ;
#6983=CARTESIAN_POINT ( 'NONE',  ( 5.000000000000003553, -20.00000000000000000, -9.999999999999994671 ) ) ;
#6996=VERTEX_POINT ( 'NONE', #16631 ) ;
#7001=DIRECTION ( 'NONE',  ( -9.858538378746663627E-23, 5.031452844637890958E-23, -1.000000000000000000 ) ) ;
#7042=DIRECTION ( 'NONE',  ( -0.9768494444668812671, -0.2139279384389642935, 0.000000000000000000 ) ) ;
#7064=VECTOR ( 'NONE', #9390, 1000.000000000000000 ) ;
#7067=ORIENTED_EDGE ( 'NONE', *, *, #12208, .F. ) ;
#7135=DIRECTION ( 'NONE',  ( 0.7969485188038759604, 0.6040472319084893016, -1.134471691914156900E-16 ) ) ;
#7144=VERTEX_POINT ( 'NONE', #12966 ) ;
#7153=AXIS2_PLACEMENT_3D ( 'NONE', #14687, #7438, #1564 ) ;
#7176=AXIS2_PLACEMENT_3D ( 'NONE', #19212, #1726, #4944 ) ;
#7188=VERTEX_POINT ( 'NONE', #17305 ) ;
#7197=LINE ( 'NONE', #2712, #11787 ) ;
#7198=ORIENTED_EDGE ( 'NONE', *, *, #17743, .T. ) ;
#7211=EDGE_CURVE ( 'NONE', #9761, #7384, #9415, .T. ) ;
#7220=EDGE_LOOP ( 'NONE', ( #18713, #3528, #18449, #12607, #8310, #11150, #9153, #1346 ) ) ;
#7227=AXIS2_PLACEMENT_3D ( 'NONE', #8759, #16325, #16618 ) ;
#7248=ORIENTED_EDGE ( 'NONE', *, *, #2696, .F. ) ;
#7251=VERTEX_POINT ( 'NONE', #8065 ) ;
#7266=CARTESIAN_POINT ( 'NONE',  ( 3.734041964264196878, -16.98388816369253362, -9.999999999999994671 ) ) ;
#7279=DIRECTION ( 'NONE',  ( 1.000000000000000000, -1.734723475976807341E-16, 0.000000000000000000 ) ) ;
#7295=EDGE_LOOP ( 'NONE', ( #18594, #12238, #18039, #19184 ) ) ;
#7305=DIRECTION ( 'NONE',  ( -0.7581610723493046322, -0.6520673188974834833, 1.125475972357111981E-16 ) ) ;
#7313=DIRECTION ( 'NONE',  ( -9.858538378746663627E-23, 5.031452844637890958E-23, -1.000000000000000000 ) ) ;
#7316=LINE ( 'NONE', #5650, #14988 ) ;
#7325=LINE ( 'NONE', #19220, #16044 ) ;
#7346=DIRECTION ( 'NONE',  ( 9.710251638871371392E-17, 5.969973981896233748E-17, 1.000000000000000000 ) ) ;
#7384=VERTEX_POINT ( 'NONE', #4559 ) ;
#7394=EDGE_LOOP ( 'NONE', ( #6639, #7439, #19080, #2167 ) ) ;
#7399=PLANE ( 'NONE',  #10713 ) ;
#7427=AXIS2_PLACEMENT_3D ( 'NONE', #8302, #967, #9962 ) ;
#7429=CARTESIAN_POINT ( 'NONE',  ( -20.00000000000000000, -19.99999999999999289, -23.00000000000000000 ) ) ;
#7438=DIRECTION ( 'NONE',  ( -9.858538378746663627E-23, 5.031452844637890958E-23, -1.000000000000000000 ) ) ;
#7439=ORIENTED_EDGE ( 'NONE', *, *, #1620, .T. ) ;
#7457=CARTESIAN_POINT ( 'NONE',  ( 2.449293598294706513E-15, -20.00000000000000000, 9.000000000000000000 ) ) ;
#7488=ORIENTED_EDGE ( 'NONE', *, *, #18257, .T. ) ;
#7524=DIRECTION ( 'NONE',  ( 0.000000000000000000, 0.000000000000000000, -1.000000000000000000 ) ) ;
#7538=ORIENTED_EDGE ( 'NONE', *, *, #7211, .T. ) ;
#7547=ADVANCED_FACE ( 'NONE', ( #2297 ), #6487, .T. ) ;
#7558=DIRECTION ( 'NONE',  ( -9.858538378746663627E-23, 5.031452844637890958E-23, -1.000000000000000000 ) ) ;
#7560=EDGE_LOOP ( 'NONE', ( #2059, #6529, #11689, #4455 ) ) ;
#7561=CARTESIAN_POINT ( 'NONE',  ( 5.000000000000003553, -20.00000000000000000, 15.00000000000000355 ) ) ;
#7583=CARTESIAN_POINT ( 'NONE',  ( 3.734041964264196878, -16.98388816369253362, -8.999999999999996447 ) ) ;
#7589=CARTESIAN_POINT ( 'NONE',  ( -20.00000000000000000, -19.99999999999999289, -20.00000000000000000 ) ) ;
#7593=ADVANCED_FACE ( 'NONE', ( #3656 ), #12669, .T. ) ;
#7602=EDGE_CURVE ( 'NONE', #3326, #9351, #5120, .T. ) ;
#7605=VERTEX_POINT ( 'NONE', #3645 ) ;
#7623=ORIENTED_EDGE ( 'NONE', *, *, #11758, .T. ) ;
#7640=EDGE_CURVE ( 'NONE', #15612, #9304, #1465, .T. ) ;
#7641=DIRECTION ( 'NONE',  ( -0.000000000000000000, -0.000000000000000000, -1.000000000000000000 ) ) ;
#7649=PLANE ( 'NONE',  #19062 ) ;
#7668=CIRCLE ( 'NONE', #2370, 15.00000000000000000 ) ;
#7681=DIRECTION ( 'NONE',  ( -1.000000000000000000, 0.000000000000000000, 0.000000000000000000 ) ) ;
#7692=ADVANCED_FACE ( 'NONE', ( #4841 ), #10802, .T. ) ;
#7693=CARTESIAN_POINT ( 'NONE',  ( 14.14213562373095101, -25.00000000000000711, -50.00000000000000000 ) ) ;
#7699=ORIENTED_EDGE ( 'NONE', *, *, #7640, .T. ) ;
#7716=ORIENTED_EDGE ( 'NONE', *, *, #8061, .F. ) ;
#7729=EDGE_CURVE ( 'NONE', #16659, #3811, #218, .T. ) ;
#7758=CARTESIAN_POINT ( 'NONE',  ( 2.449293598294706513E-15, -20.00000000000000000, -8.999999999999998224 ) ) ;
#7767=EDGE_CURVE ( 'NONE', #17357, #15934, #17296, .T. ) ;
#7798=ORIENTED_EDGE ( 'NONE', *, *, #1065, .T. ) ;
#7807=VECTOR ( 'NONE', #18303, 1000.000000000000000 ) ;
#7825=DIRECTION ( 'NONE',  ( 1.000000000000000000, -1.734723475976807341E-16, -0.000000000000000000 ) ) ;
#7843=EDGE_CURVE ( 'NONE', #18140, #16659, #6474, .T. ) ;
#7858=EDGE_CURVE ( 'NONE', #13420, #8876, #12424, .T. ) ;
#7866=VECTOR ( 'NONE', #13397, 1000.000000000000000 ) ;
#7874=DIRECTION ( 'NONE',  ( -0.000000000000000000, -0.000000000000000000, 1.000000000000000000 ) ) ;
#7878=LINE ( 'NONE', #2097, #2773 ) ;
#7887=ORIENTED_EDGE ( 'NONE', *, *, #8658, .F. ) ;
#7890=PLANE ( 'NONE',  #1874 ) ;
#7941=AXIS2_PLACEMENT_3D ( 'NONE', #8746, #17301, #1109 ) ;
#7944=EDGE_CURVE ( 'NONE', #2791, #1433, #13059, .T. ) ;
#7945=LINE ( 'NONE', #14113, #17784 ) ;
#7951=CYLINDRICAL_SURFACE ( 'NONE', #2764, 4.800000000000000711 ) ;
#7955=EDGE_CURVE ( 'NONE', #8262, #7251, #3240, .T. ) ;
#7960=CARTESIAN_POINT ( 'NONE',  ( -14.14213562373094568, -25.00000000000000000, -20.00000000000000000 ) ) ;
#7962=DIRECTION ( 'NONE',  ( -0.000000000000000000, -0.000000000000000000, -1.000000000000000000 ) ) ;
#7963=DIRECTION ( 'NONE',  ( -1.000000000000000000, 0.000000000000000000, 0.000000000000000000 ) ) ;
#7973=VECTOR ( 'NONE', #5798, 1000.000000000000000 ) ;
#7977=ORIENTED_EDGE ( 'NONE', *, *, #7767, .T. ) ;
#7990=CARTESIAN_POINT ( 'NONE',  ( 2.449293598294706513E-15, -20.00000000000000000, 9.000000000000000000 ) ) ;
#8004=DIRECTION ( 'NONE',  ( 0.000000000000000000, 0.000000000000000000, -1.000000000000000000 ) ) ;
#8005=ORIENTED_EDGE ( 'NONE', *, *, #7767, .F. ) ;
#8045=CARTESIAN_POINT ( 'NONE',  ( 1.000000000000000444, -15.10102051443364246, 9.000000000000000000 ) ) ;
#8047=DIRECTION ( 'NONE',  ( -1.000000000000000000, 0.000000000000000000, 0.000000000000000000 ) ) ;
#8048=VECTOR ( 'NONE', #171, 1000.000000000000000 ) ;
#8050=EDGE_CURVE ( 'NONE', #5143, #15934, #17460, .T. ) ;
#8056=CARTESIAN_POINT ( 'NONE',  ( -14.99999999999999822, -19.99999999999999645, -23.00000000000000000 ) ) ;
#8061=EDGE_CURVE ( 'NONE', #15612, #19390, #5170, .T. ) ;
#8065=CARTESIAN_POINT ( 'NONE',  ( 20.00000000000000000, -14.99999999999999289, -23.00000000000000000 ) ) ;
#8078=AXIS2_PLACEMENT_3D ( 'NONE', #10969, #16978, #5094 ) ;
#8085=PLANE ( 'NONE',  #15416 ) ;
#8101=VERTEX_POINT ( 'NONE', #8110 ) ;
#8105=EDGE_LOOP ( 'NONE', ( #8653, #7977, #11759, #17968 ) ) ;
#8110=CARTESIAN_POINT ( 'NONE',  ( -17.85000000000000142, -19.99999999999999289, -23.00000000000000000 ) ) ;
#8169=ORIENTED_EDGE ( 'NONE', *, *, #6754, .T. ) ;
#8209=ADVANCED_FACE ( 'NONE', ( #2834 ), #19320, .F. ) ;
#8215=AXIS2_PLACEMENT_3D ( 'NONE', #7589, #12191, #7681 ) ;
#8227=ORIENTED_EDGE ( 'NONE', *, *, #11434, .T. ) ;
#8229=DIRECTION ( 'NONE',  ( -1.000000000000000000, 0.000000000000000000, 0.000000000000000000 ) ) ;
#8251=CARTESIAN_POINT ( 'NONE',  ( -20.00000000000000000, -19.99999999999999289, -23.00000000000000000 ) ) ;
#8260=AXIS2_PLACEMENT_3D ( 'NONE', #7758, #9416, #9316 ) ;
#8262=VERTEX_POINT ( 'NONE', #19120 ) ;
#8265=ORIENTED_EDGE ( 'NONE', *, *, #16517, .T. ) ;
#8280=AXIS2_PLACEMENT_3D ( 'NONE', #17907, #143, #53 ) ;
#8302=CARTESIAN_POINT ( 'NONE',  ( 1.267864665251833278E-11, -20.00000000000000000, 9.000000000000000000 ) ) ;
#8308=EDGE_CURVE ( 'NONE', #6920, #4928, #2553, .T. ) ;
#8309=EDGE_CURVE ( 'NONE', #18696, #8779, #6194, .T. ) ;
#8310=ORIENTED_EDGE ( 'NONE', *, *, #15693, .F. ) ;
#8316=DIRECTION ( 'NONE',  ( -1.000000000000000000, 1.734723475976806848E-16, 0.000000000000000000 ) ) ;
#8362=FACE_OUTER_BOUND ( 'NONE', #11445, .T. ) ;
#8392=ORIENTED_EDGE ( 'NONE', *, *, #3820, .F. ) ;
#8404=( GEOMETRIC_REPRESENTATION_CONTEXT ( 3 ) GLOBAL_UNCERTAINTY_ASSIGNED_CONTEXT ( ( #9109 ) ) GLOBAL_UNIT_ASSIGNED_CONTEXT ( ( #18621, #2139, #4885 ) ) REPRESENTATION_CONTEXT ( 'NONE', 'WORKASPACE' ) );
#8415=ORIENTED_EDGE ( 'NONE', *, *, #301, .F. ) ;
#8427=EDGE_CURVE ( 'NONE', #9042, #3326, #3125, .T. ) ;
#8441=AXIS2_PLACEMENT_3D ( 'NONE', #2687, #4331, #8639 ) ;
#8457=CARTESIAN_POINT ( 'NONE',  ( 20.00000000000000000, -14.99999999999999289, -23.00000000000000000 ) ) ;
#8495=ORIENTED_EDGE ( 'NONE', *, *, #4360, .F. ) ;
#8506=CYLINDRICAL_SURFACE ( 'NONE', #9887, 15.00000000000000000 ) ;
#8514=DIRECTION ( 'NONE',  ( 0.000000000000000000, 0.000000000000000000, -1.000000000000000000 ) ) ;
#8516=CARTESIAN_POINT ( 'NONE',  ( 22.14999999999999858, -20.00000000000000000, -23.00000000000000000 ) ) ;
#8539=DIRECTION ( 'NONE',  ( -0.000000000000000000, -0.000000000000000000, -1.000000000000000000 ) ) ;
#8572=ADVANCED_FACE ( 'NONE', ( #9841 ), #2426, .F. ) ;
#8573=EDGE_LOOP ( 'NONE', ( #8415, #13227 ) ) ;
#8582=AXIS2_PLACEMENT_3D ( 'NONE', #7429, #7524, #3026 ) ;
#8597=VERTEX_POINT ( 'NONE', #16045 ) ;
#8616=ORIENTED_EDGE ( 'NONE', *, *, #15670, .F. ) ;
#8635=ORIENTED_EDGE ( 'NONE', *, *, #4734, .F. ) ;
#8639=DIRECTION ( 'NONE',  ( 1.000000000000000000, 0.000000000000000000, 0.000000000000000000 ) ) ;
#8651=APPLICATION_CONTEXT ( 'automotive_design' ) ;
#8653=ORIENTED_EDGE ( 'NONE', *, *, #13461, .F. ) ;
#8656=ORIENTED_EDGE ( 'NONE', *, *, #5000, .F. ) ;
#8658=EDGE_CURVE ( 'NONE', #16221, #2254, #18106, .T. ) ;
#8668=ADVANCED_FACE ( 'NONE', ( #4364 ), #18995, .F. ) ;
#8679=AXIS2_PLACEMENT_3D ( 'NONE', #476, #10671, #18248 ) ;
#8687=LINE ( 'NONE', #12010, #3737 ) ;
#8692=LINE ( 'NONE', #73, #15975 ) ;
#8695=ORIENTED_EDGE ( 'NONE', *, *, #2763, .T. ) ;
#8700=CARTESIAN_POINT ( 'NONE',  ( 2.899426713160750069, -23.82535289025860337, -8.999999999999996447 ) ) ;
#8722=CARTESIAN_POINT ( 'NONE',  ( 2.449293598294706513E-15, -20.00000000000000000, -23.00000000000000000 ) ) ;
#8730=DIRECTION ( 'NONE',  ( 1.000000000000000000, 0.000000000000000000, -0.000000000000000000 ) ) ;
#8735=CARTESIAN_POINT ( 'NONE',  ( 1.267864665261691752E-11, -20.00000000000000000, 9.999999999999998224 ) ) ;
#8742=DIRECTION ( 'NONE',  ( -1.000000000000000000, 0.000000000000000000, 0.000000000000000000 ) ) ;
#8744=DIRECTION ( 'NONE',  ( -0.2439756946365075896, 0.9697813467099857254, 1.610118993450814692E-22 ) ) ;
#8746=CARTESIAN_POINT ( 'NONE',  ( 20.00000000000000000, -20.00000000000000000, -23.00000000000000000 ) ) ;
#8759=CARTESIAN_POINT ( 'NONE',  ( 20.00000000000000000, -20.00000000000000000, -20.00000000000000000 ) ) ;
#8779=VERTEX_POINT ( 'NONE', #3278 ) ;
#8781=ORIENTED_EDGE ( 'NONE', *, *, #9024, .T. ) ;
#8795=ADVANCED_FACE ( 'NONE', ( #9158 ), #12192, .F. ) ;
#8814=LINE ( 'NONE', #10374, #9657 ) ;
#8833=DIRECTION ( 'NONE',  ( 0.000000000000000000, 0.000000000000000000, 1.000000000000000000 ) ) ;
#8834=DIRECTION ( 'NONE',  ( 0.000000000000000000, 0.000000000000000000, 1.000000000000000000 ) ) ;
#8858=FACE_BOUND ( 'NONE', #15980, .T. ) ;
#8876=VERTEX_POINT ( 'NONE', #4933 ) ;
#8902=LINE ( 'NONE', #5975, #4656 ) ;
#8953=DIRECTION ( 'NONE',  ( -1.000000000000000000, 0.000000000000000000, 0.000000000000000000 ) ) ;
#8971=ORIENTED_EDGE ( 'NONE', *, *, #8308, .F. ) ;
#8975=FACE_OUTER_BOUND ( 'NONE', #14631, .T. ) ;
#8983=CIRCLE ( 'NONE', #13362, 2.149999999999999023 ) ;
#9016=CARTESIAN_POINT ( 'NONE',  ( -4.688877333428352223, -21.02685410450703074, 9.999999999999998224 ) ) ;
#9022=CIRCLE ( 'NONE', #5275, 4.800000000000000711 ) ;
#9023=CARTESIAN_POINT ( 'NONE',  ( 2.482347295856823136E-15, -20.00000000000000000, -8.999999999999996447 ) ) ;
#9024=EDGE_CURVE ( 'NONE', #7144, #10315, #9220, .T. ) ;
#9042=VERTEX_POINT ( 'NONE', #8045 ) ;
#9043=ADVANCED_FACE ( 'NONE', ( #6231 ), #607, .T. ) ;
#9056=FACE_OUTER_BOUND ( 'NONE', #13804, .T. ) ;
#9064=LINE ( 'NONE', #531, #7807 ) ;
#9067=CYLINDRICAL_SURFACE ( 'NONE', #7176, 2.149999999999999023 ) ;
#9094=DIRECTION ( 'NONE',  ( -0.000000000000000000, -0.000000000000000000, -1.000000000000000000 ) ) ;
#9109=UNCERTAINTY_MEASURE_WITH_UNIT (LENGTH_MEASURE( 1.000000000000000082E-05 ), #18621, 'distance_accuracy_value', 'NONE');
#9143=EDGE_CURVE ( 'NONE', #12835, #7144, #2775, .T. ) ;
#9150=EDGE_CURVE ( 'NONE', #4903, #17705, #10172, .T. ) ;
#9153=ORIENTED_EDGE ( 'NONE', *, *, #1130, .F. ) ;
#9158=FACE_OUTER_BOUND ( 'NONE', #12033, .T. ) ;
#9176=EDGE_CURVE ( 'NONE', #6411, #17357, #11749, .T. ) ;
#9204=LINE ( 'NONE', #480, #7064 ) ;
#9209=DIRECTION ( 'NONE',  ( 9.858538378746663627E-23, -5.031452844637890958E-23, 1.000000000000000000 ) ) ;
#9212=CARTESIAN_POINT ( 'NONE',  ( 2.899426713160750069, -23.82535289025860337, -9.999999999999994671 ) ) ;
#9220=CIRCLE ( 'NONE', #4550, 5.000000000000000888 ) ;
#9221=DIRECTION ( 'NONE',  ( -0.000000000000000000, -0.000000000000000000, 1.000000000000000000 ) ) ;
#9234=LINE ( 'NONE', #12283, #3447 ) ;
#9251=CARTESIAN_POINT ( 'NONE',  ( 20.00000000000000000, -14.99999999999999289, -20.00000000000000000 ) ) ;
#9280=FACE_BOUND ( 'NONE', #4063, .T. ) ;
#9286=EDGE_LOOP ( 'NONE', ( #15930, #9459, #284, #8635, #2014, #5983, #11401, #16225 ) ) ;
#9290=LINE ( 'NONE', #15279, #2246 ) ;
#9303=AXIS2_PLACEMENT_3D ( 'NONE', #2650, #8514, #14484 ) ;
#9304=VERTEX_POINT ( 'NONE', #7561 ) ;
#9314=CARTESIAN_POINT ( 'NONE',  ( -1.000000000000000000, -14.00000000000000000, -9.000000000000001776 ) ) ;
#9316=DIRECTION ( 'NONE',  ( -1.000000000000000000, 0.000000000000000000, 0.000000000000000000 ) ) ;
#9327=ORIENTED_EDGE ( 'NONE', *, *, #1065, .F. ) ;
#9346=LINE ( 'NONE', #9251, #9981 ) ;
#9351=VERTEX_POINT ( 'NONE', #16690 ) ;
#9376=EDGE_LOOP ( 'NONE', ( #16985, #11950, #9828, #7067 ) ) ;
#9390=DIRECTION ( 'NONE',  ( -0.000000000000000000, -0.000000000000000000, 1.000000000000000000 ) ) ;
#9415=CIRCLE ( 'NONE', #15071, 5.000000000000000888 ) ;
#9416=DIRECTION ( 'NONE',  ( -9.710251638871371392E-17, -5.969973981896233748E-17, -1.000000000000000000 ) ) ;
#9423=CARTESIAN_POINT ( 'NONE',  ( 1.267864665261691752E-11, -20.00000000000000000, 9.999999999999998224 ) ) ;
#9434=CARTESIAN_POINT ( 'NONE',  ( 1.000000000000002442, -20.00000000000000000, -9.000000000000001776 ) ) ;
#9435=CARTESIAN_POINT ( 'NONE',  ( 2.449293598294706513E-15, -20.00000000000000000, -50.00000000000000000 ) ) ;
#9449=DIRECTION ( 'NONE',  ( 1.000000000000000000, -1.734723475976807341E-16, -0.000000000000000000 ) ) ;
#9450=ORIENTED_EDGE ( 'NONE', *, *, #14348, .T. ) ;
#9459=ORIENTED_EDGE ( 'NONE', *, *, #7729, .F. ) ;
#9474=CARTESIAN_POINT ( 'NONE',  ( 20.00000000000000000, -20.00000000000000000, -20.00000000000000000 ) ) ;
#9478=LINE ( 'NONE', #5166, #10046 ) ;
#9492=DIRECTION ( 'NONE',  ( -0.000000000000000000, -0.000000000000000000, -1.000000000000000000 ) ) ;
#9512=DIRECTION ( 'NONE',  ( -9.858538378746663627E-23, 5.031452844637890958E-23, -1.000000000000000000 ) ) ;
#9526=DIRECTION ( 'NONE',  ( -0.7779254092217071648, -0.6283566325640553840, 0.000000000000000000 ) ) ;
#9544=EDGE_CURVE ( 'NONE', #1321, #10552, #2056, .T. ) ;
#9569=ORIENTED_EDGE ( 'NONE', *, *, #18283, .T. ) ;
#9572=ORIENTED_EDGE ( 'NONE', *, *, #883, .F. ) ;
#9578=DIRECTION ( 'NONE',  ( -9.710251638871371392E-17, -5.969973981896234981E-17, -1.000000000000000000 ) ) ;
#9589=PLANE ( 'NONE',  #13778 ) ;
#9598=DIRECTION ( 'NONE',  ( -1.000000000000000000, 0.000000000000000000, 0.000000000000000000 ) ) ;
#9612=AXIS2_PLACEMENT_3D ( 'NONE', #10328, #14548, #12988 ) ;
#9614=EDGE_CURVE ( 'NONE', #10315, #5073, #2569, .T. ) ;
#9634=EDGE_LOOP ( 'NONE', ( #6365, #12125, #14607, #8971 ) ) ;
#9657=VECTOR ( 'NONE', #14786, 1000.000000000000000 ) ;
#9663=DIRECTION ( 'NONE',  ( 9.710251638871371392E-17, 5.969973981896233748E-17, 1.000000000000000000 ) ) ;
#9673=DIRECTION ( 'NONE',  ( -0.000000000000000000, -0.000000000000000000, -1.000000000000000000 ) ) ;
#9677=DIRECTION ( 'NONE',  ( 1.000000000000000000, 0.000000000000000000, 0.000000000000000000 ) ) ;
#9678=AXIS2_PLACEMENT_3D ( 'NONE', #3797, #11514, #6721 ) ;
#9708=ORIENTED_EDGE ( 'NONE', *, *, #11929, .T. ) ;
#9716=COLOUR_RGB ( '',0.8941176470588234615, 0.8941176470588234615, 0.8941176470588234615 ) ;
#9722=CARTESIAN_POINT ( 'NONE',  ( 20.00000000000000000, -25.00000000000000711, -20.00000000000000000 ) ) ;
#9761=VERTEX_POINT ( 'NONE', #10562 ) ;
#9770=CARTESIAN_POINT ( 'NONE',  ( 2.482347295856823136E-15, -20.00000000000000000, -8.999999999999996447 ) ) ;
#9773=DIRECTION ( 'NONE',  ( 1.000000000000000000, 0.000000000000000000, 0.000000000000000000 ) ) ;
#9790=DIRECTION ( 'NONE',  ( -0.7779254092217071648, -0.6283566325640553840, 0.000000000000000000 ) ) ;
#9828=ORIENTED_EDGE ( 'NONE', *, *, #7843, .T. ) ;
#9841=FACE_OUTER_BOUND ( 'NONE', #9634, .T. ) ;
#9848=VECTOR ( 'NONE', #2172, 1000.000000000000000 ) ;
#9861=CARTESIAN_POINT ( 'NONE',  ( 2.449293598294706513E-15, -20.00000000000000000, -50.00000000000000000 ) ) ;
#9872=DIRECTION ( 'NONE',  ( 9.710251638871371392E-17, 5.969973981896233748E-17, 1.000000000000000000 ) ) ;
#9883=CARTESIAN_POINT ( 'NONE',  ( 20.00000000000000000, -25.00000000000000711, -23.00000000000000000 ) ) ;
#9887=AXIS2_PLACEMENT_3D ( 'NONE', #9861, #17638, #9773 ) ;
#9898=CARTESIAN_POINT ( 'NONE',  ( -4.999999999999998224, -20.00000000000000000, 9.999999999999998224 ) ) ;
#9912=AXIS2_PLACEMENT_3D ( 'NONE', #8700, #7135, #13113 ) ;
#9919=DIRECTION ( 'NONE',  ( -0.000000000000000000, -0.000000000000000000, -1.000000000000000000 ) ) ;
#9946=CARTESIAN_POINT ( 'NONE',  ( -14.14213562373094746, -25.00000000000000000, -23.00000000000000000 ) ) ;
#9962=DIRECTION ( 'NONE',  ( -0.9768494444668812671, -0.2139279384389642935, 0.000000000000000000 ) ) ;
#9981=VECTOR ( 'NONE', #9449, 1000.000000000000000 ) ;
#9996=CIRCLE ( 'NONE', #4992, 2.149999999999999023 ) ;
#10046=VECTOR ( 'NONE', #17146, 1000.000000000000000 ) ;
#10051=CARTESIAN_POINT ( 'NONE',  ( 22.14999999999999858, -20.00000000000000000, -23.00000000000000000 ) ) ;
#10053=VERTEX_POINT ( 'NONE', #15766 ) ;
#10063=DIRECTION ( 'NONE',  ( -1.545477659731174253E-22, 3.805888647522192075E-23, -1.000000000000000000 ) ) ;
#10087=VERTEX_POINT ( 'NONE', #11719 ) ;
#10089=PRODUCT_DEFINITION ( 'UNKNOWN', '', #16398, #11655 ) ;
#10101=DIRECTION ( 'NONE',  ( -0.000000000000000000, -0.000000000000000000, -1.000000000000000000 ) ) ;
#10102=SHAPE_REPRESENTATION_RELATIONSHIP ( 'NONE' , 'NONE' ,  #19357, #5922 ) ;
#10107=ADVANCED_FACE ( 'NONE', ( #19013 ), #8506, .T. ) ;
#10147=DIRECTION ( 'NONE',  ( -1.000000000000000000, 0.000000000000000000, 0.000000000000000000 ) ) ;
#10172=CIRCLE ( 'NONE', #16156, 5.000000000000007994 ) ;
#10219=VECTOR ( 'NONE', #9673, 1000.000000000000000 ) ;
#10224=CARTESIAN_POINT ( 'NONE',  ( 2.449293598294706513E-15, -20.00000000000000000, -9.999999999999994671 ) ) ;
#10285=CARTESIAN_POINT ( 'NONE',  ( 5.000000000000003553, -20.00000000000000000, 15.00000000000000355 ) ) ;
#10295=ORIENTED_EDGE ( 'NONE', *, *, #1179, .T. ) ;
#10315=VERTEX_POINT ( 'NONE', #11916 ) ;
#10318=DIRECTION ( 'NONE',  ( -0.7779254092217071648, -0.6283566325640553840, 0.000000000000000000 ) ) ;
#10327=PLANE ( 'NONE',  #1658 ) ;
#10328=CARTESIAN_POINT ( 'NONE',  ( 2.449293598294706513E-15, -20.00000000000000000, -23.00000000000000000 ) ) ;
#10337=ADVANCED_FACE ( 'NONE', ( #8975 ), #3212, .F. ) ;
#10356=CARTESIAN_POINT ( 'NONE',  ( 2.449293598294706513E-15, -20.00000000000000000, 9.000000000000000000 ) ) ;
#10359=AXIS2_PLACEMENT_3D ( 'NONE', #2871, #8834, #16191 ) ;
#10362=EDGE_CURVE ( 'NONE', #11836, #18140, #5850, .T. ) ;
#10366=ORIENTED_EDGE ( 'NONE', *, *, #9176, .F. ) ;
#10374=CARTESIAN_POINT ( 'NONE',  ( 20.00000000000000000, -25.00000000000000711, -23.00000000000000000 ) ) ;
#10421=CARTESIAN_POINT ( 'NONE',  ( 2.449293598294706513E-15, -20.00000000000000000, -8.999999999999998224 ) ) ;
#10487=FACE_OUTER_BOUND ( 'NONE', #6409, .T. ) ;
#10492=CYLINDRICAL_SURFACE ( 'NONE', #16302, 4.799999999999999822 ) ;
#10515=CARTESIAN_POINT ( 'NONE',  ( 1.000000000000002442, -20.00000000000000000, 8.999999999999998224 ) ) ;
#10524=EDGE_CURVE ( 'NONE', #5734, #5878, #1583, .T. ) ;
#10542=CIRCLE ( 'NONE', #6470, 5.000000000000000888 ) ;
#10552=VERTEX_POINT ( 'NONE', #733 ) ;
#10562=CARTESIAN_POINT ( 'NONE',  ( -4.999999999999998224, -20.00000000000000000, -20.00000000000000000 ) ) ;
#10585=EDGE_CURVE ( 'NONE', #12060, #1649, #11904, .T. ) ;
#10588=AXIS2_PLACEMENT_3D ( 'NONE', #9883, #12931, #8316 ) ;
#10591=EDGE_CURVE ( 'NONE', #18302, #1080, #10966, .T. ) ;
#10635=VECTOR ( 'NONE', #15194, 1000.000000000000000 ) ;
#10644=CARTESIAN_POINT ( 'NONE',  ( 2.449293598294706513E-15, -20.00000000000000000, -9.999999999999994671 ) ) ;
#10652=CARTESIAN_POINT ( 'NONE',  ( 3.260336594487419859, -23.79080536174652494, -9.999999999999994671 ) ) ;
#10661=LINE ( 'NONE', #15460, #17834 ) ;
#10671=DIRECTION ( 'NONE',  ( 0.000000000000000000, 0.000000000000000000, -1.000000000000000000 ) ) ;
#10680=LINE ( 'NONE', #16683, #10635 ) ;
#10689=CARTESIAN_POINT ( 'NONE',  ( -3.734041964264191549, -23.01611183630746638, -9.999999999999994671 ) ) ;
#10694=CARTESIAN_POINT ( 'NONE',  ( 20.00000000000000000, -20.00000000000000000, -23.00000000000000000 ) ) ;
#10713=AXIS2_PLACEMENT_3D ( 'NONE', #19397, #5935, #17906 ) ;
#10802=CYLINDRICAL_SURFACE ( 'NONE', #19021, 4.799999999999999822 ) ;
#10813=FACE_OUTER_BOUND ( 'NONE', #2893, .T. ) ;
#10819=CARTESIAN_POINT ( 'NONE',  ( 14.14213562373094923, -14.99999999999999112, -20.00000000000000000 ) ) ;
#10824=DIRECTION ( 'NONE',  ( -1.000000000000000000, 0.000000000000000000, 0.000000000000000000 ) ) ;
#10828=DIRECTION ( 'NONE',  ( -0.000000000000000000, -0.000000000000000000, -1.000000000000000000 ) ) ;
#10842=VECTOR ( 'NONE', #14226, 1000.000000000000000 ) ;
#10871=CARTESIAN_POINT ( 'NONE',  ( -1.000000000000000000, -14.00000000000000000, 8.999999999999998224 ) ) ;
#10878=ADVANCED_FACE ( 'NONE', ( #14838 ), #44, .T. ) ;
#10888=DIRECTION ( 'NONE',  ( -0.000000000000000000, -0.000000000000000000, -1.000000000000000000 ) ) ;
#10897=ORIENTED_EDGE ( 'NONE', *, *, #13111, .F. ) ;
#10913=LINE ( 'NONE', #16921, #17835 ) ;
#10917=VECTOR ( 'NONE', #17503, 1000.000000000000114 ) ;
#10949=CIRCLE ( 'NONE', #2189, 4.800000000000000711 ) ;
#10953=EDGE_CURVE ( 'NONE', #8597, #1096, #649, .T. ) ;
#10955=DIRECTION ( 'NONE',  ( 9.710251638871371392E-17, 5.969973981896233748E-17, 1.000000000000000000 ) ) ;
#10966=CIRCLE ( 'NONE', #2550, 15.00000000000000000 ) ;
#10969=CARTESIAN_POINT ( 'NONE',  ( 2.449293598294706513E-15, -20.00000000000000000, 9.999999999999998224 ) ) ;
#10995=VECTOR ( 'NONE', #9919, 1000.000000000000000 ) ;
#10996=DIRECTION ( 'NONE',  ( -1.000000000000000000, 0.000000000000000000, 0.000000000000000000 ) ) ;
#11001=DIRECTION ( 'NONE',  ( -9.710251638871371392E-17, -5.969973981896233748E-17, -1.000000000000000000 ) ) ;
#11012=CARTESIAN_POINT ( 'NONE',  ( -4.688877333428352223, -21.02685410450703074, 9.000000000000000000 ) ) ;
#11022=FACE_OUTER_BOUND ( 'NONE', #7560, .T. ) ;
#11040=FACE_OUTER_BOUND ( 'NONE', #4787, .T. ) ;
#11042=EDGE_LOOP ( 'NONE', ( #16130, #15277, #3029, #11605 ) ) ;
#11058=EDGE_LOOP ( 'NONE', ( #9572, #6631, #4040, #7716 ) ) ;
#11059=ORIENTED_EDGE ( 'NONE', *, *, #12021, .T. ) ;
#11063=LINE ( 'NONE', #16779, #926 ) ;
#11071=DIRECTION ( 'NONE',  ( -1.000000000000000000, 0.000000000000000000, 0.000000000000000000 ) ) ;
#11100=EDGE_CURVE ( 'NONE', #5525, #2254, #9478, .T. ) ;
#11142=CARTESIAN_POINT ( 'NONE',  ( -4.999999999999998224, -20.00000000000000000, 15.00000000000000355 ) ) ;
#11150=ORIENTED_EDGE ( 'NONE', *, *, #12384, .T. ) ;
#11155=AXIS2_PLACEMENT_3D ( 'NONE', #16384, #7346, #12769 ) ;
#11165=LINE ( 'NONE', #18268, #2453 ) ;
#11167=CARTESIAN_POINT ( 'NONE',  ( 2.449293598294706513E-15, -20.00000000000000000, -20.00000000000000000 ) ) ;
#11188=DIRECTION ( 'NONE',  ( 0.000000000000000000, 0.000000000000000000, -1.000000000000000000 ) ) ;
#11197=VECTOR ( 'NONE', #8539, 1000.000000000000000 ) ;
#11199=CARTESIAN_POINT ( 'NONE',  ( 2.449293598294706513E-15, -20.00000000000000000, -20.00000000000000000 ) ) ;
#11204=ORIENTED_EDGE ( 'NONE', *, *, #12280, .F. ) ;
#11240=CIRCLE ( 'NONE', #6860, 5.000000000000007994 ) ;
#11258=DIRECTION ( 'NONE',  ( -0.9768494444668813781, -0.2139279384389642935, 1.428280402115105433E-22 ) ) ;
#11259=AXIS2_PLACEMENT_3D ( 'NONE', #4765, #16724, #3285 ) ;
#11311=ORIENTED_EDGE ( 'NONE', *, *, #644, .F. ) ;
#11331=ORIENTED_EDGE ( 'NONE', *, *, #9176, .T. ) ;
#11335=PLANE ( 'NONE',  #19407 ) ;
#11401=ORIENTED_EDGE ( 'NONE', *, *, #2996, .F. ) ;
#11412=EDGE_CURVE ( 'NONE', #11822, #4387, #6237, .T. ) ;
#11421=CARTESIAN_POINT ( 'NONE',  ( 20.00000000000000000, -25.00000000000000711, -20.00000000000000000 ) ) ;
#11434=EDGE_CURVE ( 'NONE', #6154, #13316, #16647, .T. ) ;
#11445=EDGE_LOOP ( 'NONE', ( #18262, #8227, #1589, #6821 ) ) ;
#11468=ADVANCED_FACE ( 'NONE', ( #15157 ), #3302, .T. ) ;
#11480=CARTESIAN_POINT ( 'NONE',  ( 2.899426713160750069, -23.82535289025860337, -9.999999999999994671 ) ) ;
#11494=AXIS2_PLACEMENT_3D ( 'NONE', #16234, #1044, #17807 ) ;
#11513=DIRECTION ( 'NONE',  ( -1.000000000000000000, 1.734723475976807094E-16, 0.000000000000000000 ) ) ;
#11514=DIRECTION ( 'NONE',  ( 9.710251638871371392E-17, 5.969973981896233748E-17, 1.000000000000000000 ) ) ;
#11528=( GEOMETRIC_REPRESENTATION_CONTEXT ( 3 ) GLOBAL_UNCERTAINTY_ASSIGNED_CONTEXT ( ( #2856 ) ) GLOBAL_UNIT_ASSIGNED_CONTEXT ( ( #11966, #14510, #1296 ) ) REPRESENTATION_CONTEXT ( 'NONE', 'WORKASPACE' ) );
#11537=CYLINDRICAL_SURFACE ( 'NONE', #14544, 5.000000000000000888 ) ;
#11551=ADVANCED_FACE ( 'NONE', ( #11022 ), #2117, .F. ) ;
#11563=CIRCLE ( 'NONE', #14391, 15.00000000000000000 ) ;
#11569=SURFACE_SIDE_STYLE ('',( #13439 ) ) ;
#11571=CIRCLE ( 'NONE', #16607, 4.800000000000000711 ) ;
#11605=ORIENTED_EDGE ( 'NONE', *, *, #2961, .F. ) ;
#11609=EDGE_CURVE ( 'NONE', #4928, #6411, #2023, .T. ) ;
#11638=CARTESIAN_POINT ( 'NONE',  ( 1.219878473194463187, -24.84890673354692936, 9.999999999999998224 ) ) ;
#11643=ORIENTED_EDGE ( 'NONE', *, *, #8427, .T. ) ;
#11655=PRODUCT_DEFINITION_CONTEXT ( 'detailed design', #8651, 'design' ) ;
#11667=EDGE_CURVE ( 'NONE', #2621, #6553, #6616, .T. ) ;
#11684=DIRECTION ( 'NONE',  ( -1.734723475976807341E-16, -1.000000000000000000, 0.000000000000000000 ) ) ;
#11689=ORIENTED_EDGE ( 'NONE', *, *, #16220, .T. ) ;
#11719=CARTESIAN_POINT ( 'NONE',  ( -0.9999999999999995559, -15.10102051443364246, 9.000000000000000000 ) ) ;
#11734=VECTOR ( 'NONE', #6738, 1000.000000000000000 ) ;
#11736=ORIENTED_EDGE ( 'NONE', *, *, #7955, .T. ) ;
#11749=CIRCLE ( 'NONE', #19298, 4.800000000000000711 ) ;
#11757=CARTESIAN_POINT ( 'NONE',  ( 2.449293598294706513E-15, -20.00000000000000000, 15.00000000000000355 ) ) ;
#11758=EDGE_CURVE ( 'NONE', #13102, #18690, #7197, .T. ) ;
#11759=ORIENTED_EDGE ( 'NONE', *, *, #15670, .T. ) ;
#11766=VECTOR ( 'NONE', #7641, 1000.000000000000000 ) ;
#11787=VECTOR ( 'NONE', #7001, 1000.000000000000000 ) ;
#11795=LINE ( 'NONE', #17800, #226 ) ;
#11798=CARTESIAN_POINT ( 'NONE',  ( 1.000000000000000444, -15.10102051443364246, -8.999999999999998224 ) ) ;
#11821=AXIS2_PLACEMENT_3D ( 'NONE', #7457, #7558, #6186 ) ;
#11822=VERTEX_POINT ( 'NONE', #18987 ) ;
#11823=DIRECTION ( 'NONE',  ( -1.000000000000000000, 0.000000000000000000, -0.000000000000000000 ) ) ;
#11836=VERTEX_POINT ( 'NONE', #7583 ) ;
#11841=MECHANICAL_DESIGN_GEOMETRIC_PRESENTATION_REPRESENTATION('',(#12237),#11528);
#11864=DIRECTION ( 'NONE',  ( -9.858538378746663627E-23, 5.031452844637890958E-23, -1.000000000000000000 ) ) ;
#11876=CARTESIAN_POINT ( 'NONE',  ( 1.000000000000000000, -14.00000000000000000, 8.999999999999998224 ) ) ;
#11880=EDGE_LOOP ( 'NONE', ( #12278, #2141, #14478, #18015, #15057, #18846, #14270, #17147, #19228 ) ) ;
#11894=EDGE_CURVE ( 'NONE', #3326, #7144, #10542, .T. ) ;
#11896=FACE_BOUND ( 'NONE', #8573, .T. ) ;
#11902=FACE_OUTER_BOUND ( 'NONE', #14241, .T. ) ;
#11904=CIRCLE ( 'NONE', #14410, 5.000000000000000888 ) ;
#11916=CARTESIAN_POINT ( 'NONE',  ( 3.260336594487419859, -23.79080536174652494, -8.999999999999998224 ) ) ;
#11922=ORIENTED_EDGE ( 'NONE', *, *, #15190, .F. ) ;
#11924=AXIS2_PLACEMENT_3D ( 'NONE', #13090, #19099, #16435 ) ;
#11929=EDGE_CURVE ( 'NONE', #9042, #7605, #1515, .T. ) ;
#11938=ORIENTED_EDGE ( 'NONE', *, *, #9614, .F. ) ;
#11946=EDGE_LOOP ( 'NONE', ( #17838, #5240, #12418, #14953, #11331, #12587, #7488, #15826 ) ) ;
#11950=ORIENTED_EDGE ( 'NONE', *, *, #10362, .T. ) ;
#11966=( LENGTH_UNIT ( ) NAMED_UNIT ( * ) SI_UNIT ( .MILLI., .METRE. ) );
#11989=EDGE_LOOP ( 'NONE', ( #5841, #3870, #8169, #3204 ) ) ;
#12010=CARTESIAN_POINT ( 'NONE',  ( 20.00000000000000000, -25.00000000000000711, -20.00000000000000000 ) ) ;
#12012=DIRECTION ( 'NONE',  ( -1.000000000000000000, 0.000000000000000000, -0.000000000000000000 ) ) ;
#12020=DIRECTION ( 'NONE',  ( -9.710251638871371392E-17, -5.969973981896233748E-17, -1.000000000000000000 ) ) ;
#12021=EDGE_CURVE ( 'NONE', #5525, #1096, #11795, .T. ) ;
#12033=EDGE_LOOP ( 'NONE', ( #18622, #11204, #10295, #16561 ) ) ;
#12050=CARTESIAN_POINT ( 'NONE',  ( 20.00000000000000000, -14.99999999999999289, -23.00000000000000000 ) ) ;
#12051=CIRCLE ( 'NONE', #6726, 4.799999999999999822 ) ;
#12053=DIRECTION ( 'NONE',  ( 0.000000000000000000, 0.000000000000000000, -1.000000000000000000 ) ) ;
#12060=VERTEX_POINT ( 'NONE', #18671 ) ;
#12106=VERTEX_POINT ( 'NONE', #7960 ) ;
#12124=ORIENTED_EDGE ( 'NONE', *, *, #11434, .F. ) ;
#12125=ORIENTED_EDGE ( 'NONE', *, *, #16256, .F. ) ;
#12139=ORIENTED_EDGE ( 'NONE', *, *, #15500, .T. ) ;
#12141=CARTESIAN_POINT ( 'NONE',  ( 2.449293598294706513E-15, -20.00000000000000000, -9.999999999999994671 ) ) ;
#12148=EDGE_CURVE ( 'NONE', #18359, #4092, #8983, .T. ) ;
#12157=EDGE_CURVE ( 'NONE', #189, #13316, #15611, .T. ) ;
#12191=DIRECTION ( 'NONE',  ( 0.000000000000000000, 0.000000000000000000, -1.000000000000000000 ) ) ;
#12192=CYLINDRICAL_SURFACE ( 'NONE', #8280, 2.149999999999999023 ) ;
#12204=VECTOR ( 'NONE', #149, 999.9999999999998863 ) ;
#12208=EDGE_CURVE ( 'NONE', #1321, #16659, #5118, .T. ) ;
#12211=ORIENTED_EDGE ( 'NONE', *, *, #2208, .T. ) ;
#12237=STYLED_ITEM ( 'NONE', ( #6004 ), #5922 ) ;
#12238=ORIENTED_EDGE ( 'NONE', *, *, #2961, .T. ) ;
#12278=ORIENTED_EDGE ( 'NONE', *, *, #12384, .F. ) ;
#12280=EDGE_CURVE ( 'NONE', #8779, #18696, #5226, .T. ) ;
#12281=CARTESIAN_POINT ( 'NONE',  ( -20.00000000000000000, -19.99999999999999289, -23.00000000000000000 ) ) ;
#12283=CARTESIAN_POINT ( 'NONE',  ( 3.260336594487421635, -23.79080536174652494, 15.00000000000000355 ) ) ;
#12284=AXIS2_PLACEMENT_3D ( 'NONE', #6910, #1043, #19200 ) ;
#12290=DIRECTION ( 'NONE',  ( -0.000000000000000000, -0.000000000000000000, -1.000000000000000000 ) ) ;
#12326=DIRECTION ( 'NONE',  ( -1.000000000000000000, 0.000000000000000000, 0.000000000000000000 ) ) ;
#12353=DIRECTION ( 'NONE',  ( -0.000000000000000000, -0.000000000000000000, -1.000000000000000000 ) ) ;
#12384=EDGE_CURVE ( 'NONE', #17210, #12106, #1801, .T. ) ;
#12395=ORIENTED_EDGE ( 'NONE', *, *, #7211, .F. ) ;
#12396=DIRECTION ( 'NONE',  ( 0.000000000000000000, 0.000000000000000000, -1.000000000000000000 ) ) ;
#12406=DIRECTION ( 'NONE',  ( -9.858538378746663627E-23, 5.031452844637890958E-23, -1.000000000000000000 ) ) ;
#12418=ORIENTED_EDGE ( 'NONE', *, *, #16344, .T. ) ;
#12424=CIRCLE ( 'NONE', #15568, 5.000000000000000888 ) ;
#12432=CARTESIAN_POINT ( 'NONE',  ( 20.00000000000000000, -25.00000000000000711, -23.00000000000000000 ) ) ;
#12444=FACE_OUTER_BOUND ( 'NONE', #11058, .T. ) ;
#12453=FACE_OUTER_BOUND ( 'NONE', #948, .T. ) ;
#12458=CIRCLE ( 'NONE', #7153, 5.000000000000000888 ) ;
#12465=DIRECTION ( 'NONE',  ( -1.000000000000000000, 0.000000000000000000, 0.000000000000000000 ) ) ;
#12480=EDGE_LOOP ( 'NONE', ( #2209, #18574, #6775, #17529 ) ) ;
#12532=DIRECTION ( 'NONE',  ( -0.000000000000000000, -0.000000000000000000, 1.000000000000000000 ) ) ;
#12534=CARTESIAN_POINT ( 'NONE',  ( 25.00000000000000711, -20.00000000000000000, -23.00000000000000000 ) ) ;
#12583=PLANE ( 'NONE',  #11259 ) ;
#12587=ORIENTED_EDGE ( 'NONE', *, *, #13461, .T. ) ;
#12607=ORIENTED_EDGE ( 'NONE', *, *, #8658, .T. ) ;
#12628=DIRECTION ( 'NONE',  ( -0.000000000000000000, -0.000000000000000000, -1.000000000000000000 ) ) ;
#12663=DIRECTION ( 'NONE',  ( -1.000000000000000000, 0.000000000000000000, 0.000000000000000000 ) ) ;
#12669=CYLINDRICAL_SURFACE ( 'NONE', #15549, 5.000000000000007994 ) ;
#12677=ADVANCED_FACE ( 'NONE', ( #3360 ), #7951, .T. ) ;
#12702=AXIS2_PLACEMENT_3D ( 'NONE', #12432, #18439, #4986 ) ;
#12712=DIRECTION ( 'NONE',  ( -1.000000000000000000, 0.000000000000000000, -0.000000000000000000 ) ) ;
#12754=EDGE_CURVE ( 'NONE', #9304, #153, #603, .T. ) ;
#12769=DIRECTION ( 'NONE',  ( -0.7779254092217071648, -0.6283566325640553840, 0.000000000000000000 ) ) ;
#12818=ADVANCED_FACE ( 'NONE', ( #15898 ), #17282, .F. ) ;
#12835=VERTEX_POINT ( 'NONE', #1094 ) ;
#12879=CARTESIAN_POINT ( 'NONE',  ( 2.899426713160750069, -23.82535289025860337, -8.999999999999996447 ) ) ;
#12881=EDGE_CURVE ( 'NONE', #8876, #9761, #5299, .T. ) ;
#12885=CARTESIAN_POINT ( 'NONE',  ( 20.00000000000000000, -14.99999999999999289, -23.00000000000000000 ) ) ;
#12894=ORIENTED_EDGE ( 'NONE', *, *, #14771, .T. ) ;
#12931=DIRECTION ( 'NONE',  ( 1.734723475976806848E-16, 1.000000000000000000, 0.000000000000000000 ) ) ;
#12949=DIRECTION ( 'NONE',  ( -0.9768494444668812671, -0.2139279384389642935, 0.000000000000000000 ) ) ;
#12955=DIRECTION ( 'NONE',  ( -1.000000000000000000, 0.000000000000000000, 0.000000000000000000 ) ) ;
#12966=CARTESIAN_POINT ( 'NONE',  ( 5.000000000000003553, -20.00000000000000000, -8.999999999999998224 ) ) ;
#12968=CIRCLE ( 'NONE', #5145, 2.149999999999999023 ) ;
#12988=DIRECTION ( 'NONE',  ( -1.000000000000000000, 0.000000000000000000, 0.000000000000000000 ) ) ;
#12998=EDGE_CURVE ( 'NONE', #4387, #16121, #16214, .T. ) ;
#13003=ADVANCED_FACE ( 'NONE', ( #10487 ), #7649, .T. ) ;
#13006=ORIENTED_EDGE ( 'NONE', *, *, #4836, .T. ) ;
#13059=CIRCLE ( 'NONE', #8679, 15.00000000000000000 ) ;
#13075=DIRECTION ( 'NONE',  ( -1.000000000000000000, 0.000000000000000000, -0.000000000000000000 ) ) ;
#13090=CARTESIAN_POINT ( 'NONE',  ( -0.9999999999999976685, -20.00000000000000000, 8.999999999999998224 ) ) ;
#13092=ORIENTED_EDGE ( 'NONE', *, *, #15145, .T. ) ;
#13097=VECTOR ( 'NONE', #9492, 1000.000000000000000 ) ;
#13102=VERTEX_POINT ( 'NONE', #9016 ) ;
#13111=EDGE_CURVE ( 'NONE', #8262, #16221, #17482, .T. ) ;
#13113=DIRECTION ( 'NONE',  ( 0.6040472319084893016, -0.7969485188038759604, -1.107688701425240251E-17 ) ) ;
#13122=CARTESIAN_POINT ( 'NONE',  ( 2.449293598294706513E-15, -20.00000000000000000, 15.00000000000000355 ) ) ;
#13174=CARTESIAN_POINT ( 'NONE',  ( 4.688877333453707941, -18.97314589549297281, 9.000000000000000000 ) ) ;
#13193=ORIENTED_EDGE ( 'NONE', *, *, #7955, .F. ) ;
#13227=ORIENTED_EDGE ( 'NONE', *, *, #12148, .F. ) ;
#13246=DIRECTION ( 'NONE',  ( 9.858538378746663627E-23, -5.031452844637890958E-23, 1.000000000000000000 ) ) ;
#13247=EDGE_CURVE ( 'NONE', #13385, #19390, #14975, .T. ) ;
#13249=FACE_OUTER_BOUND ( 'NONE', #12480, .T. ) ;
#13257=APPLICATION_CONTEXT ( 'automotive_design' ) ;
#13316=VERTEX_POINT ( 'NONE', #13997 ) ;
#13357=EDGE_LOOP ( 'NONE', ( #14741, #5554 ) ) ;
#13362=AXIS2_PLACEMENT_3D ( 'NONE', #15417, #18477, #12465 ) ;
#13382=ORIENTED_EDGE ( 'NONE', *, *, #11100, .T. ) ;
#13385=VERTEX_POINT ( 'NONE', #16077 ) ;
#13397=DIRECTION ( 'NONE',  ( 0.000000000000000000, 0.000000000000000000, -1.000000000000000000 ) ) ;
#13420=VERTEX_POINT ( 'NONE', #17453 ) ;
#13423=CIRCLE ( 'NONE', #909, 5.000000000000007994 ) ;
#13439=SURFACE_STYLE_FILL_AREA ( #2963 ) ;
#13460=ORIENTED_EDGE ( 'NONE', *, *, #16975, .T. ) ;
#13461=EDGE_CURVE ( 'NONE', #17357, #13102, #9022, .T. ) ;
#13485=AXIS2_PLACEMENT_3D ( 'NONE', #16643, #18116, #12012 ) ;
#13500=AXIS2_PLACEMENT_3D ( 'NONE', #15128, #135, #10318 ) ;
#13510=LINE ( 'NONE', #14971, #3200 ) ;
#13528=DIRECTION ( 'NONE',  ( -1.000000000000000000, 0.000000000000000000, 0.000000000000000000 ) ) ;
#13533=AXIS2_PLACEMENT_3D ( 'NONE', #10356, #1155, #8229 ) ;
#13545=DIRECTION ( 'NONE',  ( -0.7779254092217071648, -0.6283566325640553840, 0.000000000000000000 ) ) ;
#13586=ADVANCED_FACE ( 'NONE', ( #16562 ), #14880, .T. ) ;
#13668=ORIENTED_EDGE ( 'NONE', *, *, #16344, .F. ) ;
#13687=VECTOR ( 'NONE', #7825, 1000.000000000000000 ) ;
#13725=ORIENTED_EDGE ( 'NONE', *, *, #11667, .T. ) ;
#13738=CIRCLE ( 'NONE', #14675, 4.799999999999999822 ) ;
#13769=FACE_OUTER_BOUND ( 'NONE', #16673, .T. ) ;
#13774=ORIENTED_EDGE ( 'NONE', *, *, #953, .T. ) ;
#13778=AXIS2_PLACEMENT_3D ( 'NONE', #15587, #10063, #11258 ) ;
#13801=( GEOMETRIC_REPRESENTATION_CONTEXT ( 3 ) GLOBAL_UNCERTAINTY_ASSIGNED_CONTEXT ( ( #13807 ) ) GLOBAL_UNIT_ASSIGNED_CONTEXT ( ( #4325, #1386, #19353 ) ) REPRESENTATION_CONTEXT ( 'NONE', 'WORKASPACE' ) );
#13804=EDGE_LOOP ( 'NONE', ( #5050, #11643, #19008, #7248 ) ) ;
#13807=UNCERTAINTY_MEASURE_WITH_UNIT (LENGTH_MEASURE( 1.000000000000000082E-05 ), #4325, 'distance_accuracy_value', 'NONE');
#13851=LINE ( 'NONE', #18675, #1194 ) ;
#13862=DIRECTION ( 'NONE',  ( 0.1836763462126260182, -0.9829867750086872524, -1.521953536530129242E-22 ) ) ;
#13863=ORIENTED_EDGE ( 'NONE', *, *, #12157, .T. ) ;
#13869=ORIENTED_EDGE ( 'NONE', *, *, #15988, .T. ) ;
#13907=DIRECTION ( 'NONE',  ( 9.710251638871371392E-17, 5.969973981896233748E-17, 1.000000000000000000 ) ) ;
#13952=CARTESIAN_POINT ( 'NONE',  ( 0.8816464618332836567, -24.71833652004169934, 9.999999999999998224 ) ) ;
#13962=FACE_OUTER_BOUND ( 'NONE', #3864, .T. ) ;
#13975=ORIENTED_EDGE ( 'NONE', *, *, #15500, .F. ) ;
#13987=LINE ( 'NONE', #6548, #464 ) ;
#13997=CARTESIAN_POINT ( 'NONE',  ( -14.14213562373094213, -14.99999999999998757, -23.00000000000000000 ) ) ;
#14069=DIRECTION ( 'NONE',  ( -0.9768494444668812671, -0.2139279384389642935, 0.000000000000000000 ) ) ;
#14113=CARTESIAN_POINT ( 'NONE',  ( 25.00000000000000711, -20.00000000000000000, -23.00000000000000000 ) ) ;
#14115=DIRECTION ( 'NONE',  ( -0.000000000000000000, -0.000000000000000000, -1.000000000000000000 ) ) ;
#14129=DIRECTION ( 'NONE',  ( 1.000000000000000000, -1.734723475976807341E-16, -0.000000000000000000 ) ) ;
#14131=CARTESIAN_POINT ( 'NONE',  ( 2.449293598294706513E-15, -20.00000000000000000, 15.00000000000000355 ) ) ;
#14133=DIRECTION ( 'NONE',  ( -4.082155997157844188E-16, 1.000000000000000000, 0.000000000000000000 ) ) ;
#14150=CARTESIAN_POINT ( 'NONE',  ( -20.00000000000000000, -19.99999999999999289, -20.00000000000000000 ) ) ;
#14190=ORIENTED_EDGE ( 'NONE', *, *, #8308, .T. ) ;
#14193=EDGE_CURVE ( 'NONE', #16121, #10087, #1238, .T. ) ;
#14220=DIRECTION ( 'NONE',  ( 0.000000000000000000, 0.000000000000000000, -1.000000000000000000 ) ) ;
#14225=ORIENTED_EDGE ( 'NONE', *, *, #11412, .F. ) ;
#14226=DIRECTION ( 'NONE',  ( -4.082155997157844188E-16, 1.000000000000000000, 0.000000000000000000 ) ) ;
#14240=EDGE_CURVE ( 'NONE', #14289, #10053, #9064, .T. ) ;
#14241=EDGE_LOOP ( 'NONE', ( #11922, #7798, #726, #3107 ) ) ;
#14270=ORIENTED_EDGE ( 'NONE', *, *, #14292, .F. ) ;
#14289=VERTEX_POINT ( 'NONE', #10819 ) ;
#14292=EDGE_CURVE ( 'NONE', #17705, #6154, #9346, .T. ) ;
#14294=VECTOR ( 'NONE', #2992, 1000.000000000000000 ) ;
#14338=ORIENTED_EDGE ( 'NONE', *, *, #9143, .T. ) ;
#14348=EDGE_CURVE ( 'NONE', #5734, #1464, #10913, .T. ) ;
#14391=AXIS2_PLACEMENT_3D ( 'NONE', #5307, #14220, #8047 ) ;
#14410=AXIS2_PLACEMENT_3D ( 'NONE', #4863, #2114, #10824 ) ;
#14449=DIRECTION ( 'NONE',  ( -1.734723475976807341E-16, -1.000000000000000000, 0.000000000000000000 ) ) ;
#14470=ADVANCED_FACE ( 'NONE', ( #8362 ), #17405, .F. ) ;
#14478=ORIENTED_EDGE ( 'NONE', *, *, #10953, .F. ) ;
#14484=DIRECTION ( 'NONE',  ( -1.000000000000000000, 0.000000000000000000, 0.000000000000000000 ) ) ;
#14496=CARTESIAN_POINT ( 'NONE',  ( 3.129923130707922496, -23.63917314727666152, -8.999999999999996447 ) ) ;
#14510=( NAMED_UNIT ( * ) PLANE_ANGLE_UNIT ( ) SI_UNIT ( $, .RADIAN. ) );
#14519=ORIENTED_EDGE ( 'NONE', *, *, #7602, .F. ) ;
#14523=FACE_OUTER_BOUND ( 'NONE', #18012, .T. ) ;
#14529=VERTEX_POINT ( 'NONE', #3963 ) ;
#14536=PLANE ( 'NONE',  #3128 ) ;
#14544=AXIS2_PLACEMENT_3D ( 'NONE', #3712, #12628, #6838 ) ;
#14548=DIRECTION ( 'NONE',  ( 0.000000000000000000, 0.000000000000000000, -1.000000000000000000 ) ) ;
#14567=DIRECTION ( 'NONE',  ( -1.000000000000000000, 0.000000000000000000, 0.000000000000000000 ) ) ;
#14607=ORIENTED_EDGE ( 'NONE', *, *, #11609, .F. ) ;
#14614=DIRECTION ( 'NONE',  ( -1.000000000000000000, 0.000000000000000000, 0.000000000000000000 ) ) ;
#14631=EDGE_LOOP ( 'NONE', ( #9327, #3515, #15530, #14225, #15275, #8616, #18784, #5981, #19232, #11311, #9708, #6605 ) ) ;
#14651=EDGE_CURVE ( 'NONE', #3811, #13420, #19081, .T. ) ;
#14659=DIRECTION ( 'NONE',  ( -1.000000000000000000, 1.734723475976807094E-16, 0.000000000000000000 ) ) ;
#14672=CARTESIAN_POINT ( 'NONE',  ( 1.219878473194462964, -24.84890673354692936, 15.00000000000000355 ) ) ;
#14675=AXIS2_PLACEMENT_3D ( 'NONE', #9770, #9663, #6728 ) ;
#14684=ORIENTED_EDGE ( 'NONE', *, *, #14827, .F. ) ;
#14687=CARTESIAN_POINT ( 'NONE',  ( 2.449293598294706513E-15, -20.00000000000000000, 9.999999999999998224 ) ) ;
#14713=DIRECTION ( 'NONE',  ( 9.858538378746663627E-23, -5.031452844637890958E-23, 1.000000000000000000 ) ) ;
#14715=CYLINDRICAL_SURFACE ( 'NONE', #8441, 5.000000000000007994 ) ;
#14735=DIRECTION ( 'NONE',  ( -1.000000000000000000, 0.000000000000000000, 0.000000000000000000 ) ) ;
#14741=ORIENTED_EDGE ( 'NONE', *, *, #7944, .T. ) ;
#14746=DIRECTION ( 'NONE',  ( -0.6520673188974834833, 0.7581610723493046322, 1.805535875966852419E-17 ) ) ;
#14761=ORIENTED_EDGE ( 'NONE', *, *, #12881, .F. ) ;
#14767=ORIENTED_EDGE ( 'NONE', *, *, #14193, .T. ) ;
#14771=EDGE_CURVE ( 'NONE', #5073, #6996, #11063, .T. ) ;
#14786=DIRECTION ( 'NONE',  ( -1.000000000000000000, 1.734723475976807094E-16, 0.000000000000000000 ) ) ;
#14788=DIRECTION ( 'NONE',  ( -0.6520673188974834833, 0.7581610723493047432, 1.805535875966851803E-17 ) ) ;
#14814=CARTESIAN_POINT ( 'NONE',  ( 1.267864665251833278E-11, -20.00000000000000000, 9.000000000000000000 ) ) ;
#14827=EDGE_CURVE ( 'NONE', #17459, #14529, #4904, .T. ) ;
#14836=CARTESIAN_POINT ( 'NONE',  ( 20.00000000000000000, -20.00000000000000000, -23.00000000000000000 ) ) ;
#14837=EDGE_LOOP ( 'NONE', ( #932, #3134, #421, #11059 ) ) ;
#14838=FACE_OUTER_BOUND ( 'NONE', #19067, .T. ) ;
#14880=CYLINDRICAL_SURFACE ( 'NONE', #3097, 5.000000000000000888 ) ;
#14914=ADVANCED_FACE ( 'NONE', ( #6951 ), #5577, .F. ) ;
#14953=ORIENTED_EDGE ( 'NONE', *, *, #11609, .T. ) ;
#14966=LINE ( 'NONE', #166, #6635 ) ;
#14971=CARTESIAN_POINT ( 'NONE',  ( -0.9999999999999976685, -20.00000000000000000, -9.000000000000001776 ) ) ;
#14975=CIRCLE ( 'NONE', #8078, 5.000000000000000888 ) ;
#14988=VECTOR ( 'NONE', #5750, 1000.000000000000000 ) ;
#15011=DIRECTION ( 'NONE',  ( -9.710251638871371392E-17, -5.969973981896233748E-17, -1.000000000000000000 ) ) ;
#15028=ORIENTED_EDGE ( 'NONE', *, *, #2586, .F. ) ;
#15044=EDGE_CURVE ( 'NONE', #8262, #14289, #8902, .T. ) ;
#15055=EDGE_CURVE ( 'NONE', #19390, #153, #12458, .T. ) ;
#15057=ORIENTED_EDGE ( 'NONE', *, *, #14240, .F. ) ;
#15071=AXIS2_PLACEMENT_3D ( 'NONE', #11199, #5324, #18880 ) ;
#15082=AXIS2_PLACEMENT_3D ( 'NONE', #6709, #10828, #18311 ) ;
#15083=ORIENTED_EDGE ( 'NONE', *, *, #18323, .T. ) ;
#15128=CARTESIAN_POINT ( 'NONE',  ( 2.482347295856823136E-15, -20.00000000000000000, -8.999999999999996447 ) ) ;
#15145=EDGE_CURVE ( 'NONE', #18302, #15442, #8814, .T. ) ;
#15157=FACE_OUTER_BOUND ( 'NONE', #13357, .T. ) ;
#15161=DIRECTION ( 'NONE',  ( -9.710251638871371392E-17, -5.969973981896233748E-17, -1.000000000000000000 ) ) ;
#15162=EDGE_CURVE ( 'NONE', #10053, #8597, #13423, .T. ) ;
#15176=DIRECTION ( 'NONE',  ( -0.9768494444668812671, -0.2139279384389642935, 0.000000000000000000 ) ) ;
#15190=EDGE_CURVE ( 'NONE', #10087, #1056, #10661, .T. ) ;
#15194=DIRECTION ( 'NONE',  ( -0.000000000000000000, -0.000000000000000000, 1.000000000000000000 ) ) ;
#15206=MANIFOLD_SOLID_BREP ( 'M4 Clearance Hole1', #3050 ) ;
#15223=DIRECTION ( 'NONE',  ( 0.000000000000000000, 0.000000000000000000, 1.000000000000000000 ) ) ;
#15242=ADVANCED_FACE ( 'NONE', ( #11040 ), #6533, .T. ) ;
#15248=DIRECTION ( 'NONE',  ( 0.000000000000000000, 0.000000000000000000, -1.000000000000000000 ) ) ;
#15275=ORIENTED_EDGE ( 'NONE', *, *, #16517, .F. ) ;
#15277=ORIENTED_EDGE ( 'NONE', *, *, #12208, .T. ) ;
#15278=ADVANCED_FACE ( 'NONE', ( #9280, #3991 ), #11335, .T. ) ;
#15279=CARTESIAN_POINT ( 'NONE',  ( -4.999999999999998224, -20.00000000000000000, 15.00000000000000355 ) ) ;
#15311=EDGE_CURVE ( 'NONE', #11836, #1321, #13738, .T. ) ;
#15355=CARTESIAN_POINT ( 'NONE',  ( 1.000000000000000444, -15.10102051443364246, 15.00000000000000355 ) ) ;
#15384=AXIS2_PLACEMENT_3D ( 'NONE', #5854, #15248, #11823 ) ;
#15387=VECTOR ( 'NONE', #126, 1000.000000000000000 ) ;
#15394=PRODUCT_CONTEXT ( 'NONE', #13257, 'mechanical' ) ;
#15399=CIRCLE ( 'NONE', #1376, 5.000000000000000888 ) ;
#15403=DIRECTION ( 'NONE',  ( 0.1836763462126260738, -0.9829867750086873635, -1.521953536530129477E-22 ) ) ;
#15416=AXIS2_PLACEMENT_3D ( 'NONE', #15645, #741, #839 ) ;
#15417=CARTESIAN_POINT ( 'NONE',  ( 20.00000000000000000, -20.00000000000000000, -23.00000000000000000 ) ) ;
#15437=DIRECTION ( 'NONE',  ( 0.9829867750086872524, 0.1836763462126260182, -1.475957441759982183E-22 ) ) ;
#15439=DIRECTION ( 'NONE',  ( -1.000000000000000000, 0.000000000000000000, 0.000000000000000000 ) ) ;
#15442=VERTEX_POINT ( 'NONE', #16152 ) ;
#15456=EDGE_LOOP ( 'NONE', ( #10897, #11736, #13869, #19235, #13382, #7887 ) ) ;
#15460=CARTESIAN_POINT ( 'NONE',  ( -0.9999999999999995559, -15.10102051443364246, 15.00000000000000355 ) ) ;
#15492=AXIS2_PLACEMENT_3D ( 'NONE', #3647, #18666, #6868 ) ;
#15500=EDGE_CURVE ( 'NONE', #7188, #11822, #7316, .T. ) ;
#15530=ORIENTED_EDGE ( 'NONE', *, *, #12998, .F. ) ;
#15549=AXIS2_PLACEMENT_3D ( 'NONE', #8251, #7874, #17099 ) ;
#15552=EDGE_CURVE ( 'NONE', #1096, #17210, #8687, .T. ) ;
#15568=AXIS2_PLACEMENT_3D ( 'NONE', #12141, #18149, #13528 ) ;
#15587=CARTESIAN_POINT ( 'NONE',  ( 1.267864665261691752E-11, -20.00000000000000000, 9.999999999999998224 ) ) ;
#15588=ORIENTED_EDGE ( 'NONE', *, *, #3820, .T. ) ;
#15590=AXIS2_PLACEMENT_3D ( 'NONE', #2771, #16584, #16489 ) ;
#15598=ADVANCED_FACE ( 'NONE', ( #16538 ), #9067, .F. ) ;
#15611=LINE ( 'NONE', #6312, #18705 ) ;
#15612=VERTEX_POINT ( 'NONE', #1925 ) ;
#15617=CARTESIAN_POINT ( 'NONE',  ( -0.9999999999999995559, -15.10102051443364246, -8.999999999999998224 ) ) ;
#15621=ADVANCED_FACE ( 'NONE', ( #13769 ), #7890, .F. ) ;
#15630=DIRECTION ( 'NONE',  ( -0.000000000000000000, -0.000000000000000000, -1.000000000000000000 ) ) ;
#15637=DIRECTION ( 'NONE',  ( 0.000000000000000000, 0.000000000000000000, -1.000000000000000000 ) ) ;
#15645=CARTESIAN_POINT ( 'NONE',  ( -1.000000000000000000, -14.00000000000000000, 8.999999999999998224 ) ) ;
#15670=EDGE_CURVE ( 'NONE', #15934, #18690, #2178, .T. ) ;
#15693=EDGE_CURVE ( 'NONE', #17210, #2254, #1822, .T. ) ;
#15705=CARTESIAN_POINT ( 'NONE',  ( 20.00000000000000000, -20.00000000000000000, -23.00000000000000000 ) ) ;
#15717=DIRECTION ( 'NONE',  ( -1.000000000000000000, 0.000000000000000000, 0.000000000000000000 ) ) ;
#15719=LINE ( 'NONE', #6400, #16226 ) ;
#15721=CARTESIAN_POINT ( 'NONE',  ( 3.129923130707922496, -23.63917314727666152, -8.999999999999996447 ) ) ;
#15763=CARTESIAN_POINT ( 'NONE',  ( 20.00000000000000000, -20.00000000000000000, -23.00000000000000000 ) ) ;
#15766=CARTESIAN_POINT ( 'NONE',  ( 20.00000000000000000, -14.99999999999999289, -20.00000000000000000 ) ) ;
#15826=ORIENTED_EDGE ( 'NONE', *, *, #1640, .T. ) ;
#15898=FACE_OUTER_BOUND ( 'NONE', #17048, .T. ) ;
#15905=DIRECTION ( 'NONE',  ( -9.858538378746663627E-23, 5.031452844637890958E-23, -1.000000000000000000 ) ) ;
#15915=PLANE ( 'NONE',  #5759 ) ;
#15930=ORIENTED_EDGE ( 'NONE', *, *, #14651, .F. ) ;
#15934=VERTEX_POINT ( 'NONE', #13174 ) ;
#15936=ORIENTED_EDGE ( 'NONE', *, *, #1179, .F. ) ;
#15975=VECTOR ( 'NONE', #16446, 1000.000000000000000 ) ;
#15980=EDGE_LOOP ( 'NONE', ( #18645, #17425 ) ) ;
#15988=EDGE_CURVE ( 'NONE', #7251, #6069, #11240, .T. ) ;
#16026=ORIENTED_EDGE ( 'NONE', *, *, #16256, .T. ) ;
#16034=ORIENTED_EDGE ( 'NONE', *, *, #12148, .T. ) ;
#16043=CARTESIAN_POINT ( 'NONE',  ( 2.449293598294706513E-15, -20.00000000000000000, 15.00000000000000355 ) ) ;
#16044=VECTOR ( 'NONE', #5760, 1000.000000000000000 ) ;
#16045=CARTESIAN_POINT ( 'NONE',  ( 25.00000000000000711, -20.00000000000000000, -20.00000000000000000 ) ) ;
#16059=EDGE_LOOP ( 'NONE', ( #781, #13092, #134, #13863, #8495 ) ) ;
#16075=ORIENTED_EDGE ( 'NONE', *, *, #15190, .T. ) ;
#16077=CARTESIAN_POINT ( 'NONE',  ( 0.9183817310753817909, -24.91493387504115020, 9.999999999999998224 ) ) ;
#16105=ADVANCED_FACE ( 'NONE', ( #19283, #8858, #17991, #5921 ), #14536, .F. ) ;
#16119=CIRCLE ( 'NONE', #8260, 5.000000000000000888 ) ;
#16121=VERTEX_POINT ( 'NONE', #1898 ) ;
#16130=ORIENTED_EDGE ( 'NONE', *, *, #9544, .F. ) ;
#16152=CARTESIAN_POINT ( 'NONE',  ( -20.00000000000000000, -25.00000000000000000, -23.00000000000000000 ) ) ;
#16156=AXIS2_PLACEMENT_3D ( 'NONE', #1299, #17672, #3943 ) ;
#16178=ORIENTED_EDGE ( 'NONE', *, *, #2341, .T. ) ;
#16185=CARTESIAN_POINT ( 'NONE',  ( -22.14999999999999858, -19.99999999999999289, -20.00000000000000000 ) ) ;
#16191=DIRECTION ( 'NONE',  ( 1.000000000000000000, 0.000000000000000000, 0.000000000000000000 ) ) ;
#16202=AXIS2_PLACEMENT_3D ( 'NONE', #18435, #10955, #3145 ) ;
#16214=CIRCLE ( 'NONE', #11821, 5.000000000000000888 ) ;
#16220=EDGE_CURVE ( 'NONE', #8101, #1464, #9996, .T. ) ;
#16221=VERTEX_POINT ( 'NONE', #4834 ) ;
#16225=ORIENTED_EDGE ( 'NONE', *, *, #7858, .F. ) ;
#16226=VECTOR ( 'NONE', #3475, 1000.000000000000000 ) ;
#16233=EDGE_CURVE ( 'NONE', #6154, #14289, #11563, .T. ) ;
#16234=CARTESIAN_POINT ( 'NONE',  ( 1.171083334267915221, -24.65495046420793201, 9.999999999999998224 ) ) ;
#16256=EDGE_CURVE ( 'NONE', #6411, #5143, #805, .T. ) ;
#16302=AXIS2_PLACEMENT_3D ( 'NONE', #9023, #15011, #13545 ) ;
#16325=DIRECTION ( 'NONE',  ( 0.000000000000000000, 0.000000000000000000, -1.000000000000000000 ) ) ;
#16328=ORIENTED_EDGE ( 'NONE', *, *, #12881, .T. ) ;
#16344=EDGE_CURVE ( 'NONE', #153, #4928, #18175, .T. ) ;
#16354=EDGE_LOOP ( 'NONE', ( #5724, #14338, #3417, #1639 ) ) ;
#16355=CARTESIAN_POINT ( 'NONE',  ( -14.14213562373094213, -14.99999999999998757, -50.00000000000000000 ) ) ;
#16384=CARTESIAN_POINT ( 'NONE',  ( 2.385244779468109755E-15, -20.00000000000000000, -9.999999999999994671 ) ) ;
#16396=FILL_AREA_STYLE_COLOUR ( '', #9716 ) ;
#16398=PRODUCT_DEFINITION_FORMATION_WITH_SPECIFIED_SOURCE ( 'ANY', '', #17289, .NOT_KNOWN. ) ;
#16429=DIRECTION ( 'NONE',  ( -1.000000000000000000, -4.082155997157843695E-16, 0.000000000000000000 ) ) ;
#16435=DIRECTION ( 'NONE',  ( 4.082155997157843695E-16, -1.000000000000000000, 0.000000000000000000 ) ) ;
#16446=DIRECTION ( 'NONE',  ( -0.000000000000000000, -0.000000000000000000, -1.000000000000000000 ) ) ;
#16478=DIRECTION ( 'NONE',  ( -1.000000000000000000, 0.000000000000000000, 0.000000000000000000 ) ) ;
#16489=DIRECTION ( 'NONE',  ( -1.000000000000000000, 0.000000000000000000, 0.000000000000000000 ) ) ;
#16496=ADVANCED_FACE ( 'NONE', ( #19362 ), #2777, .T. ) ;
#16517=EDGE_CURVE ( 'NONE', #18690, #11822, #10949, .T. ) ;
#16538=FACE_OUTER_BOUND ( 'NONE', #3208, .T. ) ;
#16561=ORIENTED_EDGE ( 'NONE', *, *, #301, .T. ) ;
#16562=FACE_OUTER_BOUND ( 'NONE', #879, .T. ) ;
#16581=CARTESIAN_POINT ( 'NONE',  ( 1.267864665261691752E-11, -20.00000000000000000, 9.999999999999998224 ) ) ;
#16584=DIRECTION ( 'NONE',  ( 0.000000000000000000, 0.000000000000000000, -1.000000000000000000 ) ) ;
#16589=ORIENTED_EDGE ( 'NONE', *, *, #5599, .T. ) ;
#16607=AXIS2_PLACEMENT_3D ( 'NONE', #16581, #9209, #14069 ) ;
#16618=DIRECTION ( 'NONE',  ( -1.000000000000000000, 0.000000000000000000, 0.000000000000000000 ) ) ;
#16626=DIRECTION ( 'NONE',  ( 4.082155997157843695E-16, -1.000000000000000000, 0.000000000000000000 ) ) ;
#16631=CARTESIAN_POINT ( 'NONE',  ( 3.129923130707922496, -23.63917314727666152, -9.999999999999994671 ) ) ;
#16639=ORIENTED_EDGE ( 'NONE', *, *, #15311, .T. ) ;
#16643=CARTESIAN_POINT ( 'NONE',  ( 0.000000000000000000, 0.000000000000000000, 8.999999999999998224 ) ) ;
#16647=LINE ( 'NONE', #16355, #7866 ) ;
#16659=VERTEX_POINT ( 'NONE', #10689 ) ;
#16673=EDGE_LOOP ( 'NONE', ( #19325, #12139, #1036, #191 ) ) ;
#16683=CARTESIAN_POINT ( 'NONE',  ( -14.99999999999999822, -19.99999999999999645, -50.00000000000000000 ) ) ;
#16687=SHAPE_DEFINITION_REPRESENTATION ( #19198, #19357 ) ;
#16688=CIRCLE ( 'NONE', #18890, 5.000000000000000888 ) ;
#16690=CARTESIAN_POINT ( 'NONE',  ( 1.000000000000000000, -14.00000000000000000, -9.000000000000001776 ) ) ;
#16716=FACE_OUTER_BOUND ( 'NONE', #15456, .T. ) ;
#16720=ADVANCED_FACE ( 'NONE', ( #17976 ), #10492, .T. ) ;
#16724=DIRECTION ( 'NONE',  ( 0.000000000000000000, 0.000000000000000000, -1.000000000000000000 ) ) ;
#16731=DIRECTION ( 'NONE',  ( -0.9768494444668812671, -0.2139279384389642935, 0.000000000000000000 ) ) ;
#16779=CARTESIAN_POINT ( 'NONE',  ( 3.129923130707922496, -23.63917314727666152, -8.999999999999996447 ) ) ;
#16819=ADVANCED_FACE ( 'NONE', ( #12444 ), #589, .T. ) ;
#16824=DIRECTION ( 'NONE',  ( 0.000000000000000000, 0.000000000000000000, -1.000000000000000000 ) ) ;
#16875=ORIENTED_EDGE ( 'NONE', *, *, #9024, .F. ) ;
#16887=CARTESIAN_POINT ( 'NONE',  ( -19.99999999999999289, -14.99999999999998579, -23.00000000000000000 ) ) ;
#16901=ADVANCED_FACE ( 'NONE', ( #6562 ), #9589, .T. ) ;
#16921=CARTESIAN_POINT ( 'NONE',  ( -22.14999999999999858, -19.99999999999999289, -23.00000000000000000 ) ) ;
#16952=DIRECTION ( 'NONE',  ( -9.858538378746663627E-23, 5.031452844637890958E-23, -1.000000000000000000 ) ) ;
#16968=PLANE ( 'NONE',  #12702 ) ;
#16975=EDGE_CURVE ( 'NONE', #13385, #4387, #8692, .T. ) ;
#16978=DIRECTION ( 'NONE',  ( -9.858538378746663627E-23, 5.031452844637890958E-23, -1.000000000000000000 ) ) ;
#16985=ORIENTED_EDGE ( 'NONE', *, *, #15311, .F. ) ;
#16993=DIRECTION ( 'NONE',  ( 1.000000000000000000, 0.000000000000000000, 0.000000000000000000 ) ) ;
#17048=EDGE_LOOP ( 'NONE', ( #6552, #18982, #16034, #15936 ) ) ;
#17049=CIRCLE ( 'NONE', #8582, 5.000000000000007994 ) ;
#17053=ORIENTED_EDGE ( 'NONE', *, *, #16220, .F. ) ;
#17097=CARTESIAN_POINT ( 'NONE',  ( -3.734041964264191549, -23.01611183630746638, -8.999999999999996447 ) ) ;
#17099=DIRECTION ( 'NONE',  ( 1.000000000000000000, 0.000000000000000000, 0.000000000000000000 ) ) ;
#17146=DIRECTION ( 'NONE',  ( -1.000000000000000000, 1.734723475976807094E-16, 0.000000000000000000 ) ) ;
#17147=ORIENTED_EDGE ( 'NONE', *, *, #9150, .F. ) ;
#17210=VERTEX_POINT ( 'NONE', #5390 ) ;
#17254=LINE ( 'NONE', #3911, #11734 ) ;
#17262=ORIENTED_EDGE ( 'NONE', *, *, #2095, .F. ) ;
#17263=ORIENTED_EDGE ( 'NONE', *, *, #5599, .F. ) ;
#17282=CYLINDRICAL_SURFACE ( 'NONE', #6812, 2.149999999999999023 ) ;
#17289=PRODUCT ( 'motor', 'motor', '', ( #15394 ) ) ;
#17296=LINE ( 'NONE', #2857, #2431 ) ;
#17301=DIRECTION ( 'NONE',  ( -0.000000000000000000, -0.000000000000000000, 1.000000000000000000 ) ) ;
#17305=CARTESIAN_POINT ( 'NONE',  ( 0.8816464618332836567, -24.71833652004169934, 9.999999999999998224 ) ) ;
#17344=ORIENTED_EDGE ( 'NONE', *, *, #10524, .T. ) ;
#17357=VERTEX_POINT ( 'NONE', #4212 ) ;
#17367=AXIS2_PLACEMENT_3D ( 'NONE', #9435, #11188, #7963 ) ;
#17384=CARTESIAN_POINT ( 'NONE',  ( 1.171083334267915221, -24.65495046420793201, 9.999999999999998224 ) ) ;
#17396=FACE_OUTER_BOUND ( 'NONE', #7394, .T. ) ;
#17399=DIRECTION ( 'NONE',  ( -0.000000000000000000, -0.000000000000000000, 1.000000000000000000 ) ) ;
#17405=PLANE ( 'NONE',  #1552 ) ;
#17406=EDGE_LOOP ( 'NONE', ( #18978, #7623, #8265, #13975 ) ) ;
#17425=ORIENTED_EDGE ( 'NONE', *, *, #8309, .T. ) ;
#17447=DIRECTION ( 'NONE',  ( -0.000000000000000000, -0.000000000000000000, -1.000000000000000000 ) ) ;
#17453=CARTESIAN_POINT ( 'NONE',  ( 3.020236159542449172, -23.98474259401938014, -9.999999999999994671 ) ) ;
#17459=VERTEX_POINT ( 'NONE', #6957 ) ;
#17460=CIRCLE ( 'NONE', #7427, 4.800000000000000711 ) ;
#17482=CIRCLE ( 'NONE', #15590, 15.00000000000000000 ) ;
#17503=DIRECTION ( 'NONE',  ( 0.6040472319084893016, -0.7969485188038759604, -1.107688701425240097E-17 ) ) ;
#17529=ORIENTED_EDGE ( 'NONE', *, *, #15162, .T. ) ;
#17598=CYLINDRICAL_SURFACE ( 'NONE', #7941, 5.000000000000007994 ) ;
#17601=VECTOR ( 'NONE', #6514, 1000.000000000000000 ) ;
#17612=EDGE_CURVE ( 'NONE', #16121, #1649, #9290, .T. ) ;
#17638=DIRECTION ( 'NONE',  ( -0.000000000000000000, -0.000000000000000000, 1.000000000000000000 ) ) ;
#17672=DIRECTION ( 'NONE',  ( 0.000000000000000000, 0.000000000000000000, -1.000000000000000000 ) ) ;
#17705=VERTEX_POINT ( 'NONE', #18434 ) ;
#17738=CARTESIAN_POINT ( 'NONE',  ( 1.171083334267915221, -24.65495046420793201, 9.999999999999998224 ) ) ;
#17743=EDGE_CURVE ( 'NONE', #6553, #10315, #9234, .T. ) ;
#17763=VECTOR ( 'NONE', #427, 1000.000000000000000 ) ;
#17765=VECTOR ( 'NONE', #5962, 1000.000000000000000 ) ;
#17768=CARTESIAN_POINT ( 'NONE',  ( 5.000000000000003553, -20.00000000000000000, 15.00000000000000355 ) ) ;
#17781=CARTESIAN_POINT ( 'NONE',  ( -19.99999999999999289, -14.99999999999998579, -23.00000000000000000 ) ) ;
#17784=VECTOR ( 'NONE', #9221, 1000.000000000000000 ) ;
#17800=CARTESIAN_POINT ( 'NONE',  ( 20.00000000000000000, -25.00000000000000711, -23.00000000000000000 ) ) ;
#17807=DIRECTION ( 'NONE',  ( -0.2439756946365075896, 0.9697813467099856144, 1.610118993450814692E-22 ) ) ;
#17834=VECTOR ( 'NONE', #18428, 1000.000000000000000 ) ;
#17835=VECTOR ( 'NONE', #15630, 1000.000000000000000 ) ;
#17838=ORIENTED_EDGE ( 'NONE', *, *, #13247, .T. ) ;
#17890=VECTOR ( 'NONE', #11513, 1000.000000000000000 ) ;
#17906=DIRECTION ( 'NONE',  ( -1.000000000000000000, 0.000000000000000000, -0.000000000000000000 ) ) ;
#17907=CARTESIAN_POINT ( 'NONE',  ( 20.00000000000000000, -20.00000000000000000, -23.00000000000000000 ) ) ;
#17912=PLANE ( 'NONE',  #11924 ) ;
#17930=ORIENTED_EDGE ( 'NONE', *, *, #4050, .T. ) ;
#17940=ADVANCED_FACE ( 'NONE', ( #13249 ), #14715, .T. ) ;
#17968=ORIENTED_EDGE ( 'NONE', *, *, #11758, .F. ) ;
#17976=FACE_OUTER_BOUND ( 'NONE', #9376, .T. ) ;
#17979=CARTESIAN_POINT ( 'NONE',  ( -20.00000000000000000, -19.99999999999999289, -23.00000000000000000 ) ) ;
#17991=FACE_BOUND ( 'NONE', #3891, .T. ) ;
#18012=EDGE_LOOP ( 'NONE', ( #13193, #5408, #3369, #5339 ) ) ;
#18015=ORIENTED_EDGE ( 'NONE', *, *, #15162, .F. ) ;
#18039=ORIENTED_EDGE ( 'NONE', *, *, #14651, .T. ) ;
#18106=CIRCLE ( 'NONE', #9612, 15.00000000000000000 ) ;
#18116=DIRECTION ( 'NONE',  ( 0.000000000000000000, 0.000000000000000000, -1.000000000000000000 ) ) ;
#18140=VERTEX_POINT ( 'NONE', #7266 ) ;
#18149=DIRECTION ( 'NONE',  ( -9.710251638871371392E-17, -5.969973981896233748E-17, -1.000000000000000000 ) ) ;
#18162=VECTOR ( 'NONE', #16824, 1000.000000000000000 ) ;
#18169=CIRCLE ( 'NONE', #9678, 4.799999999999999822 ) ;
#18175=CIRCLE ( 'NONE', #5624, 5.000000000000000888 ) ;
#18179=CARTESIAN_POINT ( 'NONE',  ( 20.00000000000000000, -25.00000000000000711, -23.00000000000000000 ) ) ;
#18227=DIRECTION ( 'NONE',  ( -1.000000000000000000, 0.000000000000000000, 0.000000000000000000 ) ) ;
#18248=DIRECTION ( 'NONE',  ( -1.000000000000000000, 0.000000000000000000, 0.000000000000000000 ) ) ;
#18257=EDGE_CURVE ( 'NONE', #13102, #7188, #11571, .T. ) ;
#18262=ORIENTED_EDGE ( 'NONE', *, *, #14292, .T. ) ;
#18267=CARTESIAN_POINT ( 'NONE',  ( 17.85000000000000142, -20.00000000000000000, -23.00000000000000000 ) ) ;
#18268=CARTESIAN_POINT ( 'NONE',  ( 0.8816464618332836567, -24.71833652004169934, 9.999999999999998224 ) ) ;
#18281=DIRECTION ( 'NONE',  ( -0.000000000000000000, -0.000000000000000000, -1.000000000000000000 ) ) ;
#18283=EDGE_CURVE ( 'NONE', #1433, #1080, #10680, .T. ) ;
#18302=VERTEX_POINT ( 'NONE', #9946 ) ;
#18303=DIRECTION ( 'NONE',  ( 1.000000000000000000, -1.734723475976807341E-16, -0.000000000000000000 ) ) ;
#18305=DIRECTION ( 'NONE',  ( 9.858538378746663627E-23, -5.031452844637890958E-23, 1.000000000000000000 ) ) ;
#18311=DIRECTION ( 'NONE',  ( -1.000000000000000000, 0.000000000000000000, 0.000000000000000000 ) ) ;
#18323=EDGE_CURVE ( 'NONE', #5073, #11836, #18169, .T. ) ;
#18350=AXIS2_PLACEMENT_3D ( 'NONE', #3829, #13907, #9790 ) ;
#18359=VERTEX_POINT ( 'NONE', #10051 ) ;
#18428=DIRECTION ( 'NONE',  ( -0.000000000000000000, -0.000000000000000000, -1.000000000000000000 ) ) ;
#18433=ORIENTED_EDGE ( 'NONE', *, *, #1908, .T. ) ;
#18434=CARTESIAN_POINT ( 'NONE',  ( -19.99999999999999289, -14.99999999999998579, -20.00000000000000000 ) ) ;
#18435=CARTESIAN_POINT ( 'NONE',  ( 2.385244779468109755E-15, -20.00000000000000000, -9.999999999999994671 ) ) ;
#18439=DIRECTION ( 'NONE',  ( 1.734723475976806848E-16, 1.000000000000000000, 0.000000000000000000 ) ) ;
#18445=EDGE_LOOP ( 'NONE', ( #6255, #18433, #16589, #14761 ) ) ;
#18447=DIRECTION ( 'NONE',  ( -9.710251638871371392E-17, -5.969973981896233748E-17, -1.000000000000000000 ) ) ;
#18449=ORIENTED_EDGE ( 'NONE', *, *, #2095, .T. ) ;
#18454=DIRECTION ( 'NONE',  ( -0.000000000000000000, -0.000000000000000000, -1.000000000000000000 ) ) ;
#18472=CARTESIAN_POINT ( 'NONE',  ( 2.449293598294706513E-15, -20.00000000000000000, -8.999999999999998224 ) ) ;
#18477=DIRECTION ( 'NONE',  ( -0.000000000000000000, -0.000000000000000000, -1.000000000000000000 ) ) ;
#18498=CARTESIAN_POINT ( 'NONE',  ( 1.267864665251833278E-11, -20.00000000000000000, 9.000000000000000000 ) ) ;
#18527=EDGE_CURVE ( 'NONE', #6553, #6996, #19301, .T. ) ;
#18543=PLANE ( 'NONE',  #1729 ) ;
#18574=ORIENTED_EDGE ( 'NONE', *, *, #15988, .F. ) ;
#18594=ORIENTED_EDGE ( 'NONE', *, *, #18926, .F. ) ;
#18621=( LENGTH_UNIT ( ) NAMED_UNIT ( * ) SI_UNIT ( .MILLI., .METRE. ) );
#18622=ORIENTED_EDGE ( 'NONE', *, *, #4749, .F. ) ;
#18625=ORIENTED_EDGE ( 'NONE', *, *, #13111, .T. ) ;
#18645=ORIENTED_EDGE ( 'NONE', *, *, #12280, .T. ) ;
#18666=DIRECTION ( 'NONE',  ( -0.000000000000000000, -0.000000000000000000, 1.000000000000000000 ) ) ;
#18671=CARTESIAN_POINT ( 'NONE',  ( 3.020236159542449172, -23.98474259401938014, -8.999999999999998224 ) ) ;
#18675=CARTESIAN_POINT ( 'NONE',  ( 17.85000000000000142, -20.00000000000000000, -23.00000000000000000 ) ) ;
#18690=VERTEX_POINT ( 'NONE', #11012 ) ;
#18696=VERTEX_POINT ( 'NONE', #244 ) ;
#18705=VECTOR ( 'NONE', #14129, 1000.000000000000000 ) ;
#18713=ORIENTED_EDGE ( 'NONE', *, *, #18283, .F. ) ;
#18765=CARTESIAN_POINT ( 'NONE',  ( 20.00000000000000000, -20.00000000000000000, -20.00000000000000000 ) ) ;
#18770=ADVANCED_FACE ( 'NONE', ( #10813 ), #12583, .T. ) ;
#18784=ORIENTED_EDGE ( 'NONE', *, *, #8050, .F. ) ;
#18796=ORIENTED_EDGE ( 'NONE', *, *, #15044, .F. ) ;
#18829=VECTOR ( 'NONE', #18881, 1000.000000000000114 ) ;
#18831=LINE ( 'NONE', #8516, #2683 ) ;
#18846=ORIENTED_EDGE ( 'NONE', *, *, #16233, .F. ) ;
#18873=LINE ( 'NONE', #18967, #557 ) ;
#18880=DIRECTION ( 'NONE',  ( 1.000000000000000000, 0.000000000000000000, 0.000000000000000000 ) ) ;
#18881=DIRECTION ( 'NONE',  ( 0.6040472319084893016, -0.7969485188038759604, -1.107688701425240097E-17 ) ) ;
#18890=AXIS2_PLACEMENT_3D ( 'NONE', #7990, #12406, #5349 ) ;
#18926=EDGE_CURVE ( 'NONE', #10552, #12060, #6891, .T. ) ;
#18960=DIRECTION ( 'NONE',  ( -9.858538378746663627E-23, 5.031452844637890958E-23, -1.000000000000000000 ) ) ;
#18967=CARTESIAN_POINT ( 'NONE',  ( 1.171083334267915221, -24.65495046420793201, 9.000000000000000000 ) ) ;
#18978=ORIENTED_EDGE ( 'NONE', *, *, #18257, .F. ) ;
#18982=ORIENTED_EDGE ( 'NONE', *, *, #4749, .T. ) ;
#18987=CARTESIAN_POINT ( 'NONE',  ( 0.8816464618332836567, -24.71833652004169934, 9.000000000000000000 ) ) ;
#18995=PLANE ( 'NONE',  #6798 ) ;
#19008=ORIENTED_EDGE ( 'NONE', *, *, #7602, .T. ) ;
#19013=FACE_OUTER_BOUND ( 'NONE', #7220, .T. ) ;
#19021=AXIS2_PLACEMENT_3D ( 'NONE', #5029, #11001, #9526 ) ;
#19045=AXIS2_PLACEMENT_3D ( 'NONE', #5407, #809, #12955 ) ;
#19062=AXIS2_PLACEMENT_3D ( 'NONE', #11757, #8833, #8730 ) ;
#19063=DIRECTION ( 'NONE',  ( -0.9768494444668812671, -0.2139279384389642935, 0.000000000000000000 ) ) ;
#19067=EDGE_LOOP ( 'NONE', ( #3607, #2348, #12894, #484 ) ) ;
#19080=ORIENTED_EDGE ( 'NONE', *, *, #10953, .T. ) ;
#19081=LINE ( 'NONE', #9212, #10917 ) ;
#19099=DIRECTION ( 'NONE',  ( -1.000000000000000000, -4.082155997157843695E-16, 0.000000000000000000 ) ) ;
#19120=CARTESIAN_POINT ( 'NONE',  ( 14.14213562373094923, -14.99999999999999112, -23.00000000000000000 ) ) ;
#19184=ORIENTED_EDGE ( 'NONE', *, *, #4836, .F. ) ;
#19198=PRODUCT_DEFINITION_SHAPE ( 'NONE', 'NONE',  #10089 ) ;
#19200=DIRECTION ( 'NONE',  ( -1.000000000000000000, 0.000000000000000000, 0.000000000000000000 ) ) ;
#19212=CARTESIAN_POINT ( 'NONE',  ( -20.00000000000000000, -19.99999999999999289, -23.00000000000000000 ) ) ;
#19220=CARTESIAN_POINT ( 'NONE',  ( 20.00000000000000000, -14.99999999999999289, -23.00000000000000000 ) ) ;
#19228=ORIENTED_EDGE ( 'NONE', *, *, #6754, .F. ) ;
#19232=ORIENTED_EDGE ( 'NONE', *, *, #2763, .F. ) ;
#19235=ORIENTED_EDGE ( 'NONE', *, *, #787, .T. ) ;
#19259=CIRCLE ( 'NONE', #17367, 15.00000000000000000 ) ;
#19268=CARTESIAN_POINT ( 'NONE',  ( -14.99999999999999822, -19.99999999999999645, -50.00000000000000000 ) ) ;
#19283=FACE_BOUND ( 'NONE', #4382, .T. ) ;
#19298=AXIS2_PLACEMENT_3D ( 'NONE', #8735, #13246, #12949 ) ;
#19301=LINE ( 'NONE', #19402, #12204 ) ;
#19320=PLANE ( 'NONE',  #9912 ) ;
#19325=ORIENTED_EDGE ( 'NONE', *, *, #1640, .F. ) ;
#19329=DIRECTION ( 'NONE',  ( -1.000000000000000000, 0.000000000000000000, 0.000000000000000000 ) ) ;
#19353=( NAMED_UNIT ( * ) SI_UNIT ( $, .STERADIAN. ) SOLID_ANGLE_UNIT ( ) );
#19357=SHAPE_REPRESENTATION ( 'motor', ( #10359 ), #13801 ) ;
#19362=FACE_OUTER_BOUND ( 'NONE', #17406, .T. ) ;
#19390=VERTEX_POINT ( 'NONE', #9898 ) ;
#19397=CARTESIAN_POINT ( 'NONE',  ( 20.00000000000000000, -20.00000000000000000, -23.00000000000000000 ) ) ;
#19402=CARTESIAN_POINT ( 'NONE',  ( 3.129923130707922496, -23.63917314727666152, -9.999999999999994671 ) ) ;
#19407=AXIS2_PLACEMENT_3D ( 'NONE', #15763, #2342, #12712 ) ;
#19476=COLOUR_RGB('Off White',0.89,0.88,0.83);
#19477=FILL_AREA_STYLE_COLOUR('',#19476);
#19478=FILL_AREA_STYLE('',(#19477));
#19479=SURFACE_STYLE_FILL_AREA(#19478);
#19480=SURFACE_SIDE_STYLE('',(#19479));
#19481=SURFACE_STYLE_USAGE(.BOTH.,#19480);
#19482=PRESENTATION_STYLE_ASSIGNMENT((#19481));
ENDSEC;
END-ISO-10303-21;
